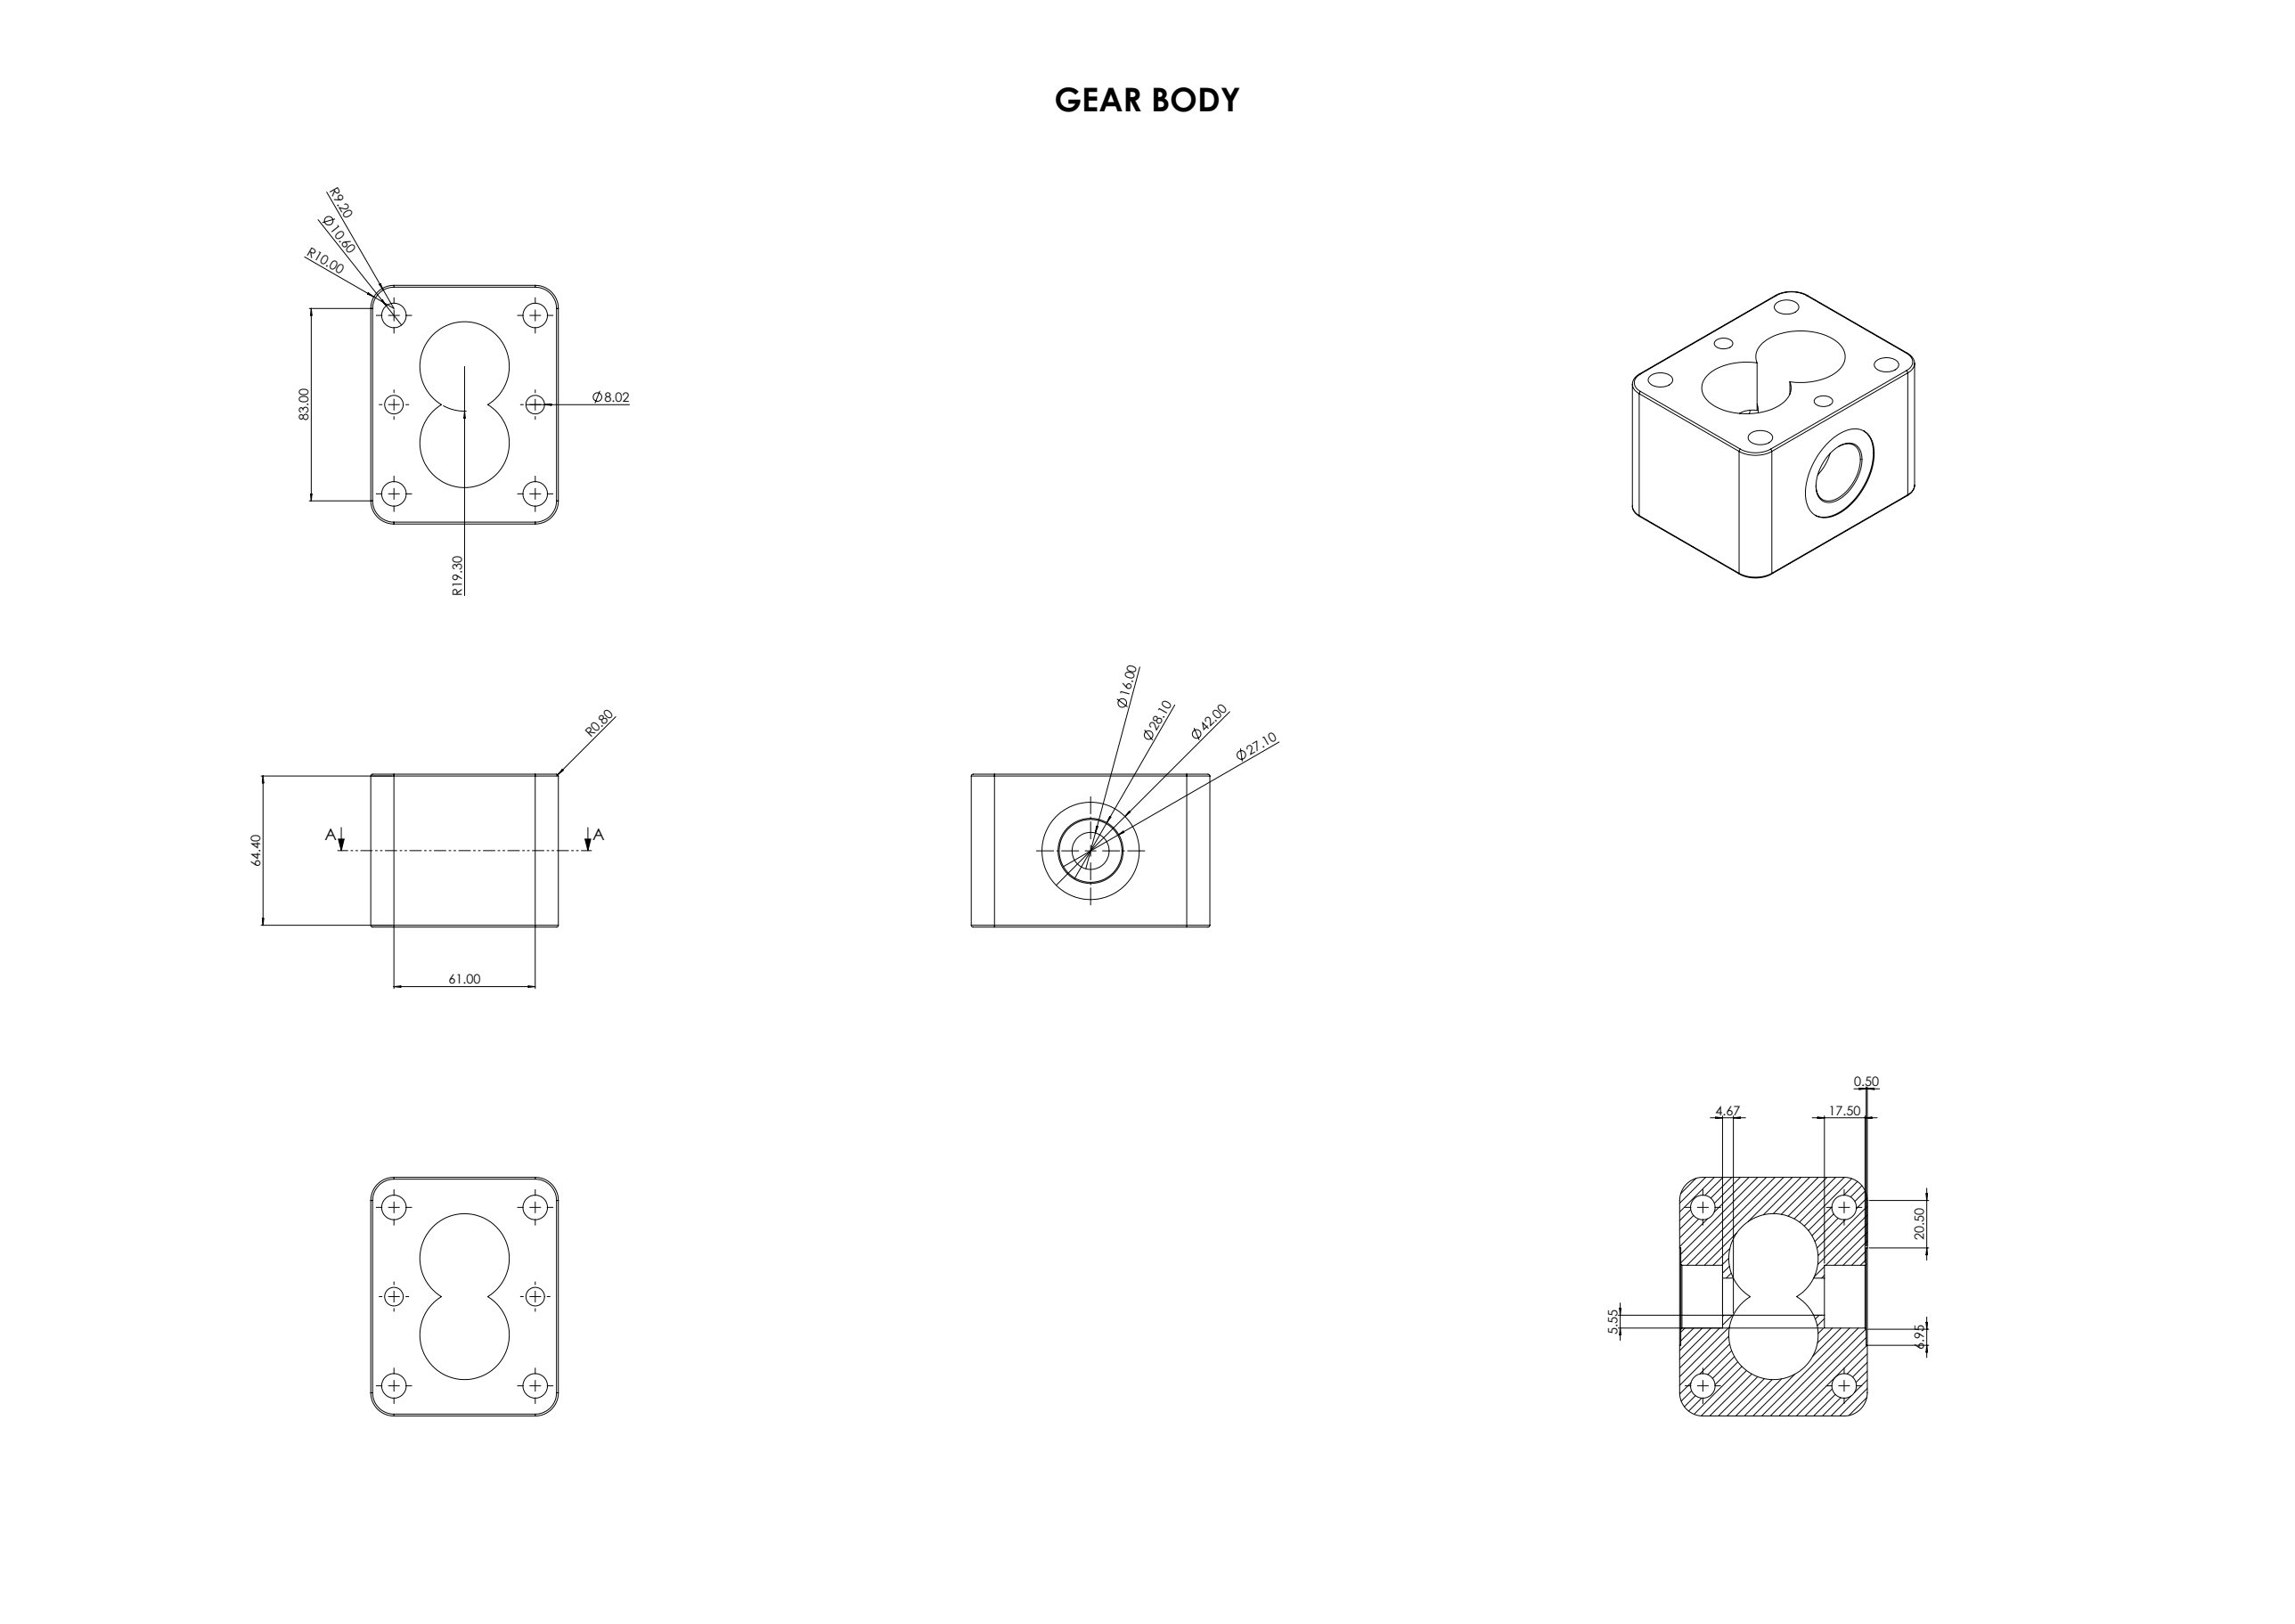
ISO-10303-21;
HEADER;
/* Generated by software containing ST-Developer
 * from STEP Tools, Inc. (www.steptools.com) 
 */

FILE_DESCRIPTION(
/* description */ (''),
/* implementation_level */ '2;1');

FILE_NAME(
/* name */ '02_Gear_Body.step',
/* time_stamp */ '2026-10-26T06:59:52-07:00',
/* author */ (''),
/* organization */ (''),
/* preprocessor_version */ 'ST-DEVELOPER v20.2',
/* originating_system */ 'Autodesk Translation Framework v15.15.0.0',
/* authorisation */ '');

FILE_SCHEMA (('AUTOMOTIVE_DESIGN { 1 0 10303 214 3 1 1 }'));
ENDSEC;

DATA;
#10=MECHANICAL_DESIGN_GEOMETRIC_PRESENTATION_REPRESENTATION('',(#165),#46395);
#137=SHAPE_REPRESENTATION_RELATIONSHIP('SRR','None',#46457,#151);
#151=ADVANCED_BREP_SHAPE_REPRESENTATION('',(#179),#46382);
#165=STYLED_ITEM('',(#46575),#179);
#179=MANIFOLD_SOLID_BREP('Body1',#24938);
#225=TOROIDAL_SURFACE('',#25463,9.19999999999999,0.8);
#226=TOROIDAL_SURFACE('',#25469,9.19999999999999,0.8);
#227=TOROIDAL_SURFACE('',#25475,9.2,0.8);
#228=TOROIDAL_SURFACE('',#25481,9.19999999999999,0.8);
#229=TOROIDAL_SURFACE('',#25503,9.19999999999999,0.8);
#230=TOROIDAL_SURFACE('',#25509,9.2,0.8);
#231=TOROIDAL_SURFACE('',#25515,9.19999999999999,0.8);
#232=TOROIDAL_SURFACE('',#25520,9.19999999999999,0.8);
#291=B_SPLINE_CURVE_WITH_KNOTS('',3,(#35527,#35528,#35529,#35530,#35531,
#35532,#35533,#35534,#35535,#35536,#35537,#35538,#35539,#35540),
 .UNSPECIFIED.,.F.,.F.,(4,2,2,2,2,2,4),(1.13912969187458,1.42739793020419,
1.87192783187775,2.07475703542203,2.27758623896631,2.45971948034335,2.64185272172039),
 .UNSPECIFIED.);
#292=B_SPLINE_CURVE_WITH_KNOTS('',3,(#35542,#35543,#35544,#35545,#35546,
#35547,#35548,#35549,#35550,#35551,#35552,#35553,#35554,#35555,#35556,#35557,
#35558,#35559,#35560,#35561,#35562,#35563,#35564,#35565,#35566,#35567),
 .UNSPECIFIED.,.F.,.F.,(4,2,2,2,2,2,2,2,2,2,2,2,4),(1.13912969187458,1.42739793020419,
1.87192783187775,2.07475703542203,2.27758623896631,2.45971948034335,2.64185272172039,
2.82398596309744,3.00611920447448,3.20894840801876,3.41177761156304,3.8563075132366,
4.14457575156621),.UNSPECIFIED.);
#293=B_SPLINE_CURVE_WITH_KNOTS('',3,(#35568,#35569,#35570,#35571,#35572,
#35573,#35574,#35575,#35576,#35577,#35578,#35579,#35580,#35581),
 .UNSPECIFIED.,.F.,.F.,(4,2,2,2,2,2,4),(2.64185272172039,2.82398596309744,
3.00611920447448,3.20894840801876,3.41177761156304,3.8563075132366,4.14457575156621),
 .UNSPECIFIED.);
#294=B_SPLINE_CURVE_WITH_KNOTS('',3,(#35587,#35588,#35589,#35590,#35591,
#35592,#35593,#35594,#35595,#35596,#35597,#35598,#35599,#35600),
 .UNSPECIFIED.,.F.,.F.,(4,2,2,2,2,2,4),(1.13912969187458,1.42739793020419,
1.87192783187775,2.07475703542203,2.27758623896631,2.45971948034335,2.64185272172039),
 .UNSPECIFIED.);
#295=B_SPLINE_CURVE_WITH_KNOTS('',3,(#35602,#35603,#35604,#35605,#35606,
#35607,#35608,#35609,#35610,#35611,#35612,#35613,#35614,#35615),
 .UNSPECIFIED.,.F.,.F.,(4,2,2,2,2,2,4),(2.64185272172039,2.82398596309744,
3.00611920447448,3.20894840801876,3.41177761156304,3.8563075132366,4.14457575156621),
 .UNSPECIFIED.);
#296=B_SPLINE_CURVE_WITH_KNOTS('',3,(#35627,#35628,#35629,#35630,#35631,
#35632,#35633,#35634,#35635,#35636,#35637,#35638,#35639,#35640,#35641,#35642,
#35643,#35644,#35645,#35646,#35647,#35648,#35649,#35650,#35651,#35652),
 .UNSPECIFIED.,.F.,.F.,(4,2,2,2,2,2,2,2,2,2,2,2,4),(1.13912969187458,1.42739793020419,
1.87192783187775,2.07475703542203,2.27758623896631,2.45971948034335,2.64185272172039,
2.82398596309744,3.00611920447448,3.20894840801876,3.41177761156304,3.8563075132366,
4.14457575156621),.UNSPECIFIED.);
#466=CYLINDRICAL_SURFACE('',#25449,13.55);
#467=CYLINDRICAL_SURFACE('',#25456,13.55);
#468=CYLINDRICAL_SURFACE('',#25460,0.8);
#469=CYLINDRICAL_SURFACE('',#25467,0.8);
#470=CYLINDRICAL_SURFACE('',#25473,0.8);
#471=CYLINDRICAL_SURFACE('',#25479,0.8);
#472=CYLINDRICAL_SURFACE('',#25484,9.99999999999999);
#473=CYLINDRICAL_SURFACE('',#25487,9.99999999999999);
#474=CYLINDRICAL_SURFACE('',#25500,0.8);
#475=CYLINDRICAL_SURFACE('',#25507,0.8);
#476=CYLINDRICAL_SURFACE('',#25513,0.8);
#477=CYLINDRICAL_SURFACE('',#25518,0.8);
#478=CYLINDRICAL_SURFACE('',#25522,10.);
#479=CYLINDRICAL_SURFACE('',#25524,9.99999999999999);
#480=CYLINDRICAL_SURFACE('',#25534,4.01);
#481=CYLINDRICAL_SURFACE('',#25537,4.01);
#482=CYLINDRICAL_SURFACE('',#25540,4.01);
#483=CYLINDRICAL_SURFACE('',#25543,4.01);
#484=CYLINDRICAL_SURFACE('',#25546,5.3);
#485=CYLINDRICAL_SURFACE('',#25547,5.3);
#486=CYLINDRICAL_SURFACE('',#25548,5.3);
#487=CYLINDRICAL_SURFACE('',#25549,5.3);
#488=CYLINDRICAL_SURFACE('',#25550,8.);
#489=CYLINDRICAL_SURFACE('',#25552,19.3);
#490=CYLINDRICAL_SURFACE('',#25554,21.);
#491=CYLINDRICAL_SURFACE('',#25556,8.);
#492=CYLINDRICAL_SURFACE('',#25558,19.3);
#493=CYLINDRICAL_SURFACE('',#25560,21.);
#611=FACE_BOUND('',#3282,.T.);
#612=FACE_BOUND('',#3286,.T.);
#613=FACE_BOUND('',#3299,.T.);
#614=FACE_BOUND('',#3301,.T.);
#615=FACE_BOUND('',#3302,.T.);
#616=FACE_BOUND('',#3303,.T.);
#617=FACE_BOUND('',#3304,.T.);
#618=FACE_BOUND('',#3305,.T.);
#619=FACE_BOUND('',#3306,.T.);
#620=FACE_BOUND('',#3307,.T.);
#621=FACE_BOUND('',#3320,.T.);
#622=FACE_BOUND('',#3321,.T.);
#623=FACE_BOUND('',#3322,.T.);
#624=FACE_BOUND('',#3323,.T.);
#625=FACE_BOUND('',#3324,.T.);
#626=FACE_BOUND('',#3325,.T.);
#627=FACE_BOUND('',#3326,.T.);
#628=FACE_BOUND('',#3342,.T.);
#629=FACE_BOUND('',#3347,.T.);
#630=FACE_BOUND('',#3350,.T.);
#764=PLANE('',#25451);
#765=PLANE('',#25458);
#766=PLANE('',#25486);
#767=PLANE('',#25489);
#768=PLANE('',#25491);
#769=PLANE('',#25523);
#770=PLANE('',#25525);
#771=PLANE('',#25536);
#772=PLANE('',#25539);
#773=PLANE('',#25542);
#774=PLANE('',#25545);
#775=PLANE('',#25553);
#776=PLANE('',#25559);
#777=PLANE('',#25561);
#1923=FACE_OUTER_BOUND('',#3279,.T.);
#1924=FACE_OUTER_BOUND('',#3280,.T.);
#1925=FACE_OUTER_BOUND('',#3281,.T.);
#1926=FACE_OUTER_BOUND('',#3283,.T.);
#1927=FACE_OUTER_BOUND('',#3284,.T.);
#1928=FACE_OUTER_BOUND('',#3285,.T.);
#1929=FACE_OUTER_BOUND('',#3287,.T.);
#1930=FACE_OUTER_BOUND('',#3288,.T.);
#1931=FACE_OUTER_BOUND('',#3289,.T.);
#1932=FACE_OUTER_BOUND('',#3290,.T.);
#1933=FACE_OUTER_BOUND('',#3291,.T.);
#1934=FACE_OUTER_BOUND('',#3292,.T.);
#1935=FACE_OUTER_BOUND('',#3293,.T.);
#1936=FACE_OUTER_BOUND('',#3294,.T.);
#1937=FACE_OUTER_BOUND('',#3295,.T.);
#1938=FACE_OUTER_BOUND('',#3296,.T.);
#1939=FACE_OUTER_BOUND('',#3297,.T.);
#1940=FACE_OUTER_BOUND('',#3298,.T.);
#1941=FACE_OUTER_BOUND('',#3300,.T.);
#1942=FACE_OUTER_BOUND('',#3308,.T.);
#1943=FACE_OUTER_BOUND('',#3309,.T.);
#1944=FACE_OUTER_BOUND('',#3310,.T.);
#1945=FACE_OUTER_BOUND('',#3311,.T.);
#1946=FACE_OUTER_BOUND('',#3312,.T.);
#1947=FACE_OUTER_BOUND('',#3313,.T.);
#1948=FACE_OUTER_BOUND('',#3314,.T.);
#1949=FACE_OUTER_BOUND('',#3315,.T.);
#1950=FACE_OUTER_BOUND('',#3316,.T.);
#1951=FACE_OUTER_BOUND('',#3317,.T.);
#1952=FACE_OUTER_BOUND('',#3318,.T.);
#1953=FACE_OUTER_BOUND('',#3319,.T.);
#1954=FACE_OUTER_BOUND('',#3327,.T.);
#1955=FACE_OUTER_BOUND('',#3328,.T.);
#1956=FACE_OUTER_BOUND('',#3329,.T.);
#1957=FACE_OUTER_BOUND('',#3330,.T.);
#1958=FACE_OUTER_BOUND('',#3331,.T.);
#1959=FACE_OUTER_BOUND('',#3332,.T.);
#1960=FACE_OUTER_BOUND('',#3333,.T.);
#1961=FACE_OUTER_BOUND('',#3334,.T.);
#1962=FACE_OUTER_BOUND('',#3335,.T.);
#1963=FACE_OUTER_BOUND('',#3336,.T.);
#1964=FACE_OUTER_BOUND('',#3337,.T.);
#1965=FACE_OUTER_BOUND('',#3338,.T.);
#1966=FACE_OUTER_BOUND('',#3339,.T.);
#1967=FACE_OUTER_BOUND('',#3340,.T.);
#1968=FACE_OUTER_BOUND('',#3341,.T.);
#1969=FACE_OUTER_BOUND('',#3343,.T.);
#1970=FACE_OUTER_BOUND('',#3344,.T.);
#1971=FACE_OUTER_BOUND('',#3345,.T.);
#1972=FACE_OUTER_BOUND('',#3346,.T.);
#1973=FACE_OUTER_BOUND('',#3348,.T.);
#1974=FACE_OUTER_BOUND('',#3349,.T.);
#3279=EDGE_LOOP('',(#17354,#17355,#17356,#17357));
#3280=EDGE_LOOP('',(#17358,#17359,#17360,#17361));
#3281=EDGE_LOOP('',(#17362));
#3282=EDGE_LOOP('',(#17363));
#3283=EDGE_LOOP('',(#17364,#17365,#17366,#17367));
#3284=EDGE_LOOP('',(#17368,#17369,#17370,#17371));
#3285=EDGE_LOOP('',(#17372));
#3286=EDGE_LOOP('',(#17373));
#3287=EDGE_LOOP('',(#17374,#17375,#17376,#17377));
#3288=EDGE_LOOP('',(#17378,#17379,#17380,#17381));
#3289=EDGE_LOOP('',(#17382,#17383,#17384,#17385));
#3290=EDGE_LOOP('',(#17386,#17387,#17388,#17389));
#3291=EDGE_LOOP('',(#17390,#17391,#17392,#17393));
#3292=EDGE_LOOP('',(#17394,#17395,#17396,#17397));
#3293=EDGE_LOOP('',(#17398,#17399,#17400,#17401));
#3294=EDGE_LOOP('',(#17402,#17403,#17404,#17405));
#3295=EDGE_LOOP('',(#17406,#17407,#17408,#17409));
#3296=EDGE_LOOP('',(#17410,#17411,#17412,#17413));
#3297=EDGE_LOOP('',(#17414,#17415,#17416,#17417));
#3298=EDGE_LOOP('',(#17418,#17419,#17420,#17421));
#3299=EDGE_LOOP('',(#17422));
#3300=EDGE_LOOP('',(#17423,#17424,#17425,#17426,#17427,#17428,#17429,#17430));
#3301=EDGE_LOOP('',(#17431));
#3302=EDGE_LOOP('',(#17432));
#3303=EDGE_LOOP('',(#17433,#17434));
#3304=EDGE_LOOP('',(#17435));
#3305=EDGE_LOOP('',(#17436));
#3306=EDGE_LOOP('',(#17437));
#3307=EDGE_LOOP('',(#17438));
#3308=EDGE_LOOP('',(#17439,#17440,#17441,#17442));
#3309=EDGE_LOOP('',(#17443,#17444,#17445,#17446));
#3310=EDGE_LOOP('',(#17447,#17448,#17449,#17450));
#3311=EDGE_LOOP('',(#17451,#17452,#17453,#17454));
#3312=EDGE_LOOP('',(#17455,#17456,#17457,#17458));
#3313=EDGE_LOOP('',(#17459,#17460,#17461,#17462));
#3314=EDGE_LOOP('',(#17463,#17464,#17465,#17466));
#3315=EDGE_LOOP('',(#17467,#17468,#17469,#17470));
#3316=EDGE_LOOP('',(#17471,#17472,#17473,#17474));
#3317=EDGE_LOOP('',(#17475,#17476,#17477,#17478));
#3318=EDGE_LOOP('',(#17479,#17480,#17481,#17482));
#3319=EDGE_LOOP('',(#17483,#17484,#17485,#17486,#17487,#17488,#17489,#17490));
#3320=EDGE_LOOP('',(#17491));
#3321=EDGE_LOOP('',(#17492));
#3322=EDGE_LOOP('',(#17493,#17494));
#3323=EDGE_LOOP('',(#17495));
#3324=EDGE_LOOP('',(#17496));
#3325=EDGE_LOOP('',(#17497));
#3326=EDGE_LOOP('',(#17498));
#3327=EDGE_LOOP('',(#17499,#17500,#17501,#17502));
#3328=EDGE_LOOP('',(#17503));
#3329=EDGE_LOOP('',(#17504,#17505,#17506,#17507));
#3330=EDGE_LOOP('',(#17508));
#3331=EDGE_LOOP('',(#17509,#17510,#17511,#17512));
#3332=EDGE_LOOP('',(#17513));
#3333=EDGE_LOOP('',(#17514,#17515,#17516,#17517));
#3334=EDGE_LOOP('',(#17518));
#3335=EDGE_LOOP('',(#17519,#17520,#17521,#17522));
#3336=EDGE_LOOP('',(#17523,#17524,#17525,#17526));
#3337=EDGE_LOOP('',(#17527,#17528,#17529,#17530));
#3338=EDGE_LOOP('',(#17531,#17532,#17533,#17534));
#3339=EDGE_LOOP('',(#17535,#17536,#17537,#17538,#17539,#17540));
#3340=EDGE_LOOP('',(#17541,#17542,#17543,#17544,#17545,#17546,#17547,#17548,
#17549,#17550));
#3341=EDGE_LOOP('',(#17551));
#3342=EDGE_LOOP('',(#17552));
#3343=EDGE_LOOP('',(#17553,#17554,#17555,#17556));
#3344=EDGE_LOOP('',(#17557,#17558,#17559,#17560,#17561,#17562));
#3345=EDGE_LOOP('',(#17563,#17564,#17565,#17566,#17567,#17568,#17569,#17570));
#3346=EDGE_LOOP('',(#17571));
#3347=EDGE_LOOP('',(#17572));
#3348=EDGE_LOOP('',(#17573,#17574,#17575,#17576));
#3349=EDGE_LOOP('',(#17577,#17578,#17579,#17580));
#3350=EDGE_LOOP('',(#17581));
#4722=LINE('',#35324,#7591);
#4723=LINE('',#35328,#7592);
#4724=LINE('',#35337,#7593);
#4725=LINE('',#35341,#7594);
#4726=LINE('',#35351,#7595);
#4727=LINE('',#35354,#7596);
#4728=LINE('',#35365,#7597);
#4729=LINE('',#35366,#7598);
#4730=LINE('',#35377,#7599);
#4731=LINE('',#35378,#7600);
#4732=LINE('',#35389,#7601);
#4733=LINE('',#35390,#7602);
#4734=LINE('',#35396,#7603);
#4735=LINE('',#35399,#7604);
#4736=LINE('',#35402,#7605);
#4737=LINE('',#35403,#7606);
#4738=LINE('',#35406,#7607);
#4739=LINE('',#35410,#7608);
#4740=LINE('',#35411,#7609);
#4741=LINE('',#35436,#7610);
#4742=LINE('',#35447,#7611);
#4743=LINE('',#35448,#7612);
#4744=LINE('',#35458,#7613);
#4745=LINE('',#35459,#7614);
#4746=LINE('',#35467,#7615);
#4747=LINE('',#35471,#7616);
#4748=LINE('',#35472,#7617);
#4749=LINE('',#35474,#7618);
#4750=LINE('',#35495,#7619);
#4751=LINE('',#35500,#7620);
#4752=LINE('',#35505,#7621);
#4753=LINE('',#35510,#7622);
#4754=LINE('',#35514,#7623);
#4755=LINE('',#35516,#7624);
#4756=LINE('',#35518,#7625);
#4757=LINE('',#35520,#7626);
#4758=LINE('',#35525,#7627);
#4759=LINE('',#35583,#7628);
#4760=LINE('',#35585,#7629);
#4761=LINE('',#35616,#7630);
#4762=LINE('',#35617,#7631);
#4763=LINE('',#35622,#7632);
#4764=LINE('',#35626,#7633);
#4765=LINE('',#35656,#7634);
#7591=VECTOR('',#27805,13.8);
#7592=VECTOR('',#27810,13.55);
#7593=VECTOR('',#27821,13.8);
#7594=VECTOR('',#27826,13.55);
#7595=VECTOR('',#27837,10.);
#7596=VECTOR('',#27840,10.);
#7597=VECTOR('',#27853,10.);
#7598=VECTOR('',#27854,10.);
#7599=VECTOR('',#27867,10.);
#7600=VECTOR('',#27868,10.);
#7601=VECTOR('',#27881,10.);
#7602=VECTOR('',#27882,10.);
#7603=VECTOR('',#27891,10.);
#7604=VECTOR('',#27894,10.);
#7605=VECTOR('',#27897,10.);
#7606=VECTOR('',#27898,10.);
#7607=VECTOR('',#27901,10.);
#7608=VECTOR('',#27906,10.);
#7609=VECTOR('',#27907,10.);
#7610=VECTOR('',#27934,10.);
#7611=VECTOR('',#27947,10.);
#7612=VECTOR('',#27948,10.);
#7613=VECTOR('',#27961,10.);
#7614=VECTOR('',#27962,10.);
#7615=VECTOR('',#27973,10.);
#7616=VECTOR('',#27980,10.);
#7617=VECTOR('',#27981,10.);
#7618=VECTOR('',#27984,10.);
#7619=VECTOR('',#28007,4.01);
#7620=VECTOR('',#28014,4.01);
#7621=VECTOR('',#28021,4.01);
#7622=VECTOR('',#28028,4.01);
#7623=VECTOR('',#28035,5.3);
#7624=VECTOR('',#28038,5.3);
#7625=VECTOR('',#28041,5.3);
#7626=VECTOR('',#28044,5.3);
#7627=VECTOR('',#28049,8.);
#7628=VECTOR('',#28052,10.);
#7629=VECTOR('',#28053,10.);
#7630=VECTOR('',#28054,10.);
#7631=VECTOR('',#28055,10.);
#7632=VECTOR('',#28062,21.);
#7633=VECTOR('',#28067,8.);
#7634=VECTOR('',#28074,21.);
#10441=CIRCLE('',#25447,14.05);
#10442=CIRCLE('',#25448,13.55);
#10443=CIRCLE('',#25450,13.55);
#10444=CIRCLE('',#25452,21.);
#10445=CIRCLE('',#25454,14.05);
#10446=CIRCLE('',#25455,13.55);
#10447=CIRCLE('',#25457,13.55);
#10448=CIRCLE('',#25459,21.);
#10449=CIRCLE('',#25461,0.800000000000001);
#10450=CIRCLE('',#25462,0.800000000000001);
#10451=CIRCLE('',#25464,0.799999999999992);
#10452=CIRCLE('',#25465,9.19999999999999);
#10453=CIRCLE('',#25466,9.99999999999999);
#10454=CIRCLE('',#25468,0.800000000000001);
#10455=CIRCLE('',#25470,0.800000000000005);
#10456=CIRCLE('',#25471,9.19999999999999);
#10457=CIRCLE('',#25472,9.99999999999999);
#10458=CIRCLE('',#25474,0.800000000000001);
#10459=CIRCLE('',#25476,0.800000000000001);
#10460=CIRCLE('',#25477,9.2);
#10461=CIRCLE('',#25478,9.99999999999999);
#10462=CIRCLE('',#25480,0.800000000000001);
#10463=CIRCLE('',#25482,9.19999999999999);
#10464=CIRCLE('',#25483,9.99999999999999);
#10465=CIRCLE('',#25485,9.99999999999999);
#10466=CIRCLE('',#25488,9.99999999999999);
#10467=CIRCLE('',#25490,21.);
#10468=CIRCLE('',#25492,4.01);
#10469=CIRCLE('',#25493,4.01);
#10470=CIRCLE('',#25494,19.3);
#10471=CIRCLE('',#25495,19.3);
#10472=CIRCLE('',#25496,5.3);
#10473=CIRCLE('',#25497,5.3);
#10474=CIRCLE('',#25498,5.3);
#10475=CIRCLE('',#25499,5.3);
#10476=CIRCLE('',#25501,0.800000000000001);
#10477=CIRCLE('',#25502,0.799999999999992);
#10478=CIRCLE('',#25504,0.800000000000001);
#10479=CIRCLE('',#25505,9.19999999999999);
#10480=CIRCLE('',#25506,9.99999999999999);
#10481=CIRCLE('',#25508,0.800000000000005);
#10482=CIRCLE('',#25510,0.799999999999996);
#10483=CIRCLE('',#25511,9.2);
#10484=CIRCLE('',#25512,9.99999999999999);
#10485=CIRCLE('',#25514,0.80000000000001);
#10486=CIRCLE('',#25516,0.800000000000001);
#10487=CIRCLE('',#25517,9.19999999999999);
#10488=CIRCLE('',#25519,0.799999999999992);
#10489=CIRCLE('',#25521,9.19999999999999);
#10490=CIRCLE('',#25526,4.01);
#10491=CIRCLE('',#25527,4.01);
#10492=CIRCLE('',#25528,19.3);
#10493=CIRCLE('',#25529,19.3);
#10494=CIRCLE('',#25530,5.3);
#10495=CIRCLE('',#25531,5.3);
#10496=CIRCLE('',#25532,5.3);
#10497=CIRCLE('',#25533,5.3);
#10498=CIRCLE('',#25535,4.01);
#10499=CIRCLE('',#25538,4.01);
#10500=CIRCLE('',#25541,4.01);
#10501=CIRCLE('',#25544,4.01);
#10502=CIRCLE('',#25551,8.);
#10503=CIRCLE('',#25555,21.);
#10504=CIRCLE('',#25557,8.);
#10984=VERTEX_POINT('',#35321);
#10985=VERTEX_POINT('',#35323);
#10986=VERTEX_POINT('',#35327);
#10987=VERTEX_POINT('',#35331);
#10988=VERTEX_POINT('',#35334);
#10989=VERTEX_POINT('',#35336);
#10990=VERTEX_POINT('',#35340);
#10991=VERTEX_POINT('',#35344);
#10992=VERTEX_POINT('',#35347);
#10993=VERTEX_POINT('',#35348);
#10994=VERTEX_POINT('',#35350);
#10995=VERTEX_POINT('',#35352);
#10996=VERTEX_POINT('',#35356);
#10997=VERTEX_POINT('',#35357);
#10998=VERTEX_POINT('',#35362);
#10999=VERTEX_POINT('',#35363);
#11000=VERTEX_POINT('',#35368);
#11001=VERTEX_POINT('',#35369);
#11002=VERTEX_POINT('',#35374);
#11003=VERTEX_POINT('',#35375);
#11004=VERTEX_POINT('',#35380);
#11005=VERTEX_POINT('',#35381);
#11006=VERTEX_POINT('',#35386);
#11007=VERTEX_POINT('',#35387);
#11008=VERTEX_POINT('',#35395);
#11009=VERTEX_POINT('',#35397);
#11010=VERTEX_POINT('',#35401);
#11011=VERTEX_POINT('',#35405);
#11012=VERTEX_POINT('',#35409);
#11013=VERTEX_POINT('',#35412);
#11014=VERTEX_POINT('',#35415);
#11015=VERTEX_POINT('',#35417);
#11016=VERTEX_POINT('',#35419);
#11017=VERTEX_POINT('',#35420);
#11018=VERTEX_POINT('',#35423);
#11019=VERTEX_POINT('',#35425);
#11020=VERTEX_POINT('',#35427);
#11021=VERTEX_POINT('',#35429);
#11022=VERTEX_POINT('',#35432);
#11023=VERTEX_POINT('',#35434);
#11024=VERTEX_POINT('',#35438);
#11025=VERTEX_POINT('',#35439);
#11026=VERTEX_POINT('',#35444);
#11027=VERTEX_POINT('',#35445);
#11028=VERTEX_POINT('',#35450);
#11029=VERTEX_POINT('',#35451);
#11030=VERTEX_POINT('',#35456);
#11031=VERTEX_POINT('',#35461);
#11032=VERTEX_POINT('',#35465);
#11033=VERTEX_POINT('',#35477);
#11034=VERTEX_POINT('',#35479);
#11035=VERTEX_POINT('',#35481);
#11036=VERTEX_POINT('',#35482);
#11037=VERTEX_POINT('',#35485);
#11038=VERTEX_POINT('',#35487);
#11039=VERTEX_POINT('',#35489);
#11040=VERTEX_POINT('',#35491);
#11041=VERTEX_POINT('',#35494);
#11042=VERTEX_POINT('',#35499);
#11043=VERTEX_POINT('',#35504);
#11044=VERTEX_POINT('',#35509);
#11045=VERTEX_POINT('',#35522);
#11046=VERTEX_POINT('',#35524);
#11047=VERTEX_POINT('',#35526);
#11048=VERTEX_POINT('',#35541);
#11049=VERTEX_POINT('',#35584);
#11050=VERTEX_POINT('',#35586);
#11051=VERTEX_POINT('',#35601);
#11052=VERTEX_POINT('',#35620);
#11053=VERTEX_POINT('',#35624);
#13430=EDGE_CURVE('',#10984,#10984,#10441,.T.);
#13431=EDGE_CURVE('',#10984,#10985,#4722,.T.);
#13432=EDGE_CURVE('',#10985,#10985,#10442,.T.);
#13433=EDGE_CURVE('',#10985,#10986,#4723,.T.);
#13434=EDGE_CURVE('',#10986,#10986,#10443,.T.);
#13435=EDGE_CURVE('',#10987,#10987,#10444,.T.);
#13436=EDGE_CURVE('',#10988,#10988,#10445,.T.);
#13437=EDGE_CURVE('',#10988,#10989,#4724,.T.);
#13438=EDGE_CURVE('',#10989,#10989,#10446,.T.);
#13439=EDGE_CURVE('',#10989,#10990,#4725,.T.);
#13440=EDGE_CURVE('',#10990,#10990,#10447,.T.);
#13441=EDGE_CURVE('',#10991,#10991,#10448,.T.);
#13442=EDGE_CURVE('',#10992,#10993,#10449,.T.);
#13443=EDGE_CURVE('',#10993,#10994,#4726,.T.);
#13444=EDGE_CURVE('',#10994,#10995,#10450,.T.);
#13445=EDGE_CURVE('',#10995,#10992,#4727,.T.);
#13446=EDGE_CURVE('',#10996,#10997,#10451,.T.);
#13447=EDGE_CURVE('',#10997,#10995,#10452,.T.);
#13448=EDGE_CURVE('',#10994,#10996,#10453,.T.);
#13449=EDGE_CURVE('',#10998,#10999,#10454,.T.);
#13450=EDGE_CURVE('',#10999,#10997,#4728,.T.);
#13451=EDGE_CURVE('',#10996,#10998,#4729,.T.);
#13452=EDGE_CURVE('',#11000,#11001,#10455,.T.);
#13453=EDGE_CURVE('',#11001,#10999,#10456,.T.);
#13454=EDGE_CURVE('',#10998,#11000,#10457,.T.);
#13455=EDGE_CURVE('',#11002,#11003,#10458,.T.);
#13456=EDGE_CURVE('',#11003,#11001,#4730,.T.);
#13457=EDGE_CURVE('',#11000,#11002,#4731,.T.);
#13458=EDGE_CURVE('',#11004,#11005,#10459,.T.);
#13459=EDGE_CURVE('',#11005,#11003,#10460,.T.);
#13460=EDGE_CURVE('',#11002,#11004,#10461,.T.);
#13461=EDGE_CURVE('',#11006,#11007,#10462,.T.);
#13462=EDGE_CURVE('',#11007,#11005,#4732,.T.);
#13463=EDGE_CURVE('',#11004,#11006,#4733,.T.);
#13464=EDGE_CURVE('',#10992,#11007,#10463,.T.);
#13465=EDGE_CURVE('',#11006,#10993,#10464,.T.);
#13466=EDGE_CURVE('',#11008,#10998,#4734,.T.);
#13467=EDGE_CURVE('',#11009,#11008,#10465,.T.);
#13468=EDGE_CURVE('',#11009,#11000,#4735,.T.);
#13469=EDGE_CURVE('',#11010,#10996,#4736,.T.);
#13470=EDGE_CURVE('',#11008,#11010,#4737,.T.);
#13471=EDGE_CURVE('',#11011,#10994,#4738,.T.);
#13472=EDGE_CURVE('',#11010,#11011,#10466,.T.);
#13473=EDGE_CURVE('',#11012,#10993,#4739,.T.);
#13474=EDGE_CURVE('',#11011,#11012,#4740,.T.);
#13475=EDGE_CURVE('',#11013,#11013,#10467,.T.);
#13476=EDGE_CURVE('',#11014,#11014,#10468,.T.);
#13477=EDGE_CURVE('',#11015,#11015,#10469,.T.);
#13478=EDGE_CURVE('',#11016,#11017,#10470,.T.);
#13479=EDGE_CURVE('',#11017,#11016,#10471,.T.);
#13480=EDGE_CURVE('',#11018,#11018,#10472,.T.);
#13481=EDGE_CURVE('',#11019,#11019,#10473,.T.);
#13482=EDGE_CURVE('',#11020,#11020,#10474,.T.);
#13483=EDGE_CURVE('',#11021,#11021,#10475,.T.);
#13484=EDGE_CURVE('',#11022,#11011,#10476,.T.);
#13485=EDGE_CURVE('',#11012,#11023,#10477,.T.);
#13486=EDGE_CURVE('',#11023,#11022,#4741,.T.);
#13487=EDGE_CURVE('',#11024,#11025,#10478,.T.);
#13488=EDGE_CURVE('',#11025,#11023,#10479,.T.);
#13489=EDGE_CURVE('',#11012,#11024,#10480,.T.);
#13490=EDGE_CURVE('',#11026,#11027,#10481,.T.);
#13491=EDGE_CURVE('',#11027,#11025,#4742,.T.);
#13492=EDGE_CURVE('',#11024,#11026,#4743,.T.);
#13493=EDGE_CURVE('',#11028,#11029,#10482,.T.);
#13494=EDGE_CURVE('',#11029,#11027,#10483,.T.);
#13495=EDGE_CURVE('',#11026,#11028,#10484,.T.);
#13496=EDGE_CURVE('',#11009,#11030,#10485,.T.);
#13497=EDGE_CURVE('',#11030,#11029,#4744,.T.);
#13498=EDGE_CURVE('',#11028,#11009,#4745,.T.);
#13499=EDGE_CURVE('',#11008,#11031,#10486,.T.);
#13500=EDGE_CURVE('',#11031,#11030,#10487,.T.);
#13501=EDGE_CURVE('',#11010,#11032,#10488,.T.);
#13502=EDGE_CURVE('',#11032,#11031,#4746,.T.);
#13503=EDGE_CURVE('',#11022,#11032,#10489,.T.);
#13504=EDGE_CURVE('',#11028,#11002,#4747,.T.);
#13505=EDGE_CURVE('',#11026,#11004,#4748,.T.);
#13506=EDGE_CURVE('',#11024,#11006,#4749,.T.);
#13507=EDGE_CURVE('',#11033,#11033,#10490,.T.);
#13508=EDGE_CURVE('',#11034,#11034,#10491,.T.);
#13509=EDGE_CURVE('',#11035,#11036,#10492,.T.);
#13510=EDGE_CURVE('',#11036,#11035,#10493,.T.);
#13511=EDGE_CURVE('',#11037,#11037,#10494,.T.);
#13512=EDGE_CURVE('',#11038,#11038,#10495,.T.);
#13513=EDGE_CURVE('',#11039,#11039,#10496,.T.);
#13514=EDGE_CURVE('',#11040,#11040,#10497,.T.);
#13515=EDGE_CURVE('',#11014,#11041,#4750,.T.);
#13516=EDGE_CURVE('',#11041,#11041,#10498,.T.);
#13517=EDGE_CURVE('',#11015,#11042,#4751,.T.);
#13518=EDGE_CURVE('',#11042,#11042,#10499,.T.);
#13519=EDGE_CURVE('',#11033,#11043,#4752,.T.);
#13520=EDGE_CURVE('',#11043,#11043,#10500,.T.);
#13521=EDGE_CURVE('',#11034,#11044,#4753,.T.);
#13522=EDGE_CURVE('',#11044,#11044,#10501,.T.);
#13523=EDGE_CURVE('',#11040,#11021,#4754,.T.);
#13524=EDGE_CURVE('',#11039,#11020,#4755,.T.);
#13525=EDGE_CURVE('',#11038,#11019,#4756,.T.);
#13526=EDGE_CURVE('',#11037,#11018,#4757,.T.);
#13527=EDGE_CURVE('',#11045,#11045,#10502,.T.);
#13528=EDGE_CURVE('',#11045,#11046,#4758,.T.);
#13529=EDGE_CURVE('',#11047,#11046,#291,.T.);
#13530=EDGE_CURVE('',#11048,#11047,#292,.T.);
#13531=EDGE_CURVE('',#11046,#11048,#293,.T.);
#13532=EDGE_CURVE('',#11048,#11017,#4759,.T.);
#13533=EDGE_CURVE('',#11049,#11016,#4760,.T.);
#13534=EDGE_CURVE('',#11049,#11050,#294,.T.);
#13535=EDGE_CURVE('',#11050,#11051,#295,.T.);
#13536=EDGE_CURVE('',#11036,#11051,#4761,.T.);
#13537=EDGE_CURVE('',#11035,#11047,#4762,.T.);
#13538=EDGE_CURVE('',#11052,#11052,#10503,.T.);
#13539=EDGE_CURVE('',#11052,#10991,#4763,.T.);
#13540=EDGE_CURVE('',#11053,#11053,#10504,.T.);
#13541=EDGE_CURVE('',#11053,#11050,#4764,.T.);
#13542=EDGE_CURVE('',#11051,#11049,#296,.T.);
#13543=EDGE_CURVE('',#11013,#10987,#4765,.T.);
#17354=ORIENTED_EDGE('',*,*,#13430,.T.);
#17355=ORIENTED_EDGE('',*,*,#13431,.T.);
#17356=ORIENTED_EDGE('',*,*,#13432,.T.);
#17357=ORIENTED_EDGE('',*,*,#13431,.F.);
#17358=ORIENTED_EDGE('',*,*,#13432,.F.);
#17359=ORIENTED_EDGE('',*,*,#13433,.T.);
#17360=ORIENTED_EDGE('',*,*,#13434,.T.);
#17361=ORIENTED_EDGE('',*,*,#13433,.F.);
#17362=ORIENTED_EDGE('',*,*,#13435,.F.);
#17363=ORIENTED_EDGE('',*,*,#13430,.F.);
#17364=ORIENTED_EDGE('',*,*,#13436,.T.);
#17365=ORIENTED_EDGE('',*,*,#13437,.T.);
#17366=ORIENTED_EDGE('',*,*,#13438,.T.);
#17367=ORIENTED_EDGE('',*,*,#13437,.F.);
#17368=ORIENTED_EDGE('',*,*,#13438,.F.);
#17369=ORIENTED_EDGE('',*,*,#13439,.T.);
#17370=ORIENTED_EDGE('',*,*,#13440,.T.);
#17371=ORIENTED_EDGE('',*,*,#13439,.F.);
#17372=ORIENTED_EDGE('',*,*,#13441,.F.);
#17373=ORIENTED_EDGE('',*,*,#13436,.F.);
#17374=ORIENTED_EDGE('',*,*,#13442,.T.);
#17375=ORIENTED_EDGE('',*,*,#13443,.T.);
#17376=ORIENTED_EDGE('',*,*,#13444,.T.);
#17377=ORIENTED_EDGE('',*,*,#13445,.T.);
#17378=ORIENTED_EDGE('',*,*,#13446,.T.);
#17379=ORIENTED_EDGE('',*,*,#13447,.T.);
#17380=ORIENTED_EDGE('',*,*,#13444,.F.);
#17381=ORIENTED_EDGE('',*,*,#13448,.T.);
#17382=ORIENTED_EDGE('',*,*,#13449,.T.);
#17383=ORIENTED_EDGE('',*,*,#13450,.T.);
#17384=ORIENTED_EDGE('',*,*,#13446,.F.);
#17385=ORIENTED_EDGE('',*,*,#13451,.T.);
#17386=ORIENTED_EDGE('',*,*,#13452,.T.);
#17387=ORIENTED_EDGE('',*,*,#13453,.T.);
#17388=ORIENTED_EDGE('',*,*,#13449,.F.);
#17389=ORIENTED_EDGE('',*,*,#13454,.T.);
#17390=ORIENTED_EDGE('',*,*,#13455,.T.);
#17391=ORIENTED_EDGE('',*,*,#13456,.T.);
#17392=ORIENTED_EDGE('',*,*,#13452,.F.);
#17393=ORIENTED_EDGE('',*,*,#13457,.T.);
#17394=ORIENTED_EDGE('',*,*,#13458,.T.);
#17395=ORIENTED_EDGE('',*,*,#13459,.T.);
#17396=ORIENTED_EDGE('',*,*,#13455,.F.);
#17397=ORIENTED_EDGE('',*,*,#13460,.T.);
#17398=ORIENTED_EDGE('',*,*,#13461,.T.);
#17399=ORIENTED_EDGE('',*,*,#13462,.T.);
#17400=ORIENTED_EDGE('',*,*,#13458,.F.);
#17401=ORIENTED_EDGE('',*,*,#13463,.T.);
#17402=ORIENTED_EDGE('',*,*,#13442,.F.);
#17403=ORIENTED_EDGE('',*,*,#13464,.T.);
#17404=ORIENTED_EDGE('',*,*,#13461,.F.);
#17405=ORIENTED_EDGE('',*,*,#13465,.T.);
#17406=ORIENTED_EDGE('',*,*,#13454,.F.);
#17407=ORIENTED_EDGE('',*,*,#13466,.F.);
#17408=ORIENTED_EDGE('',*,*,#13467,.F.);
#17409=ORIENTED_EDGE('',*,*,#13468,.T.);
#17410=ORIENTED_EDGE('',*,*,#13451,.F.);
#17411=ORIENTED_EDGE('',*,*,#13469,.F.);
#17412=ORIENTED_EDGE('',*,*,#13470,.F.);
#17413=ORIENTED_EDGE('',*,*,#13466,.T.);
#17414=ORIENTED_EDGE('',*,*,#13448,.F.);
#17415=ORIENTED_EDGE('',*,*,#13471,.F.);
#17416=ORIENTED_EDGE('',*,*,#13472,.F.);
#17417=ORIENTED_EDGE('',*,*,#13469,.T.);
#17418=ORIENTED_EDGE('',*,*,#13443,.F.);
#17419=ORIENTED_EDGE('',*,*,#13473,.F.);
#17420=ORIENTED_EDGE('',*,*,#13474,.F.);
#17421=ORIENTED_EDGE('',*,*,#13471,.T.);
#17422=ORIENTED_EDGE('',*,*,#13475,.T.);
#17423=ORIENTED_EDGE('',*,*,#13445,.F.);
#17424=ORIENTED_EDGE('',*,*,#13447,.F.);
#17425=ORIENTED_EDGE('',*,*,#13450,.F.);
#17426=ORIENTED_EDGE('',*,*,#13453,.F.);
#17427=ORIENTED_EDGE('',*,*,#13456,.F.);
#17428=ORIENTED_EDGE('',*,*,#13459,.F.);
#17429=ORIENTED_EDGE('',*,*,#13462,.F.);
#17430=ORIENTED_EDGE('',*,*,#13464,.F.);
#17431=ORIENTED_EDGE('',*,*,#13476,.T.);
#17432=ORIENTED_EDGE('',*,*,#13477,.T.);
#17433=ORIENTED_EDGE('',*,*,#13478,.T.);
#17434=ORIENTED_EDGE('',*,*,#13479,.T.);
#17435=ORIENTED_EDGE('',*,*,#13480,.T.);
#17436=ORIENTED_EDGE('',*,*,#13481,.T.);
#17437=ORIENTED_EDGE('',*,*,#13482,.T.);
#17438=ORIENTED_EDGE('',*,*,#13483,.T.);
#17439=ORIENTED_EDGE('',*,*,#13484,.T.);
#17440=ORIENTED_EDGE('',*,*,#13474,.T.);
#17441=ORIENTED_EDGE('',*,*,#13485,.T.);
#17442=ORIENTED_EDGE('',*,*,#13486,.T.);
#17443=ORIENTED_EDGE('',*,*,#13487,.T.);
#17444=ORIENTED_EDGE('',*,*,#13488,.T.);
#17445=ORIENTED_EDGE('',*,*,#13485,.F.);
#17446=ORIENTED_EDGE('',*,*,#13489,.T.);
#17447=ORIENTED_EDGE('',*,*,#13490,.T.);
#17448=ORIENTED_EDGE('',*,*,#13491,.T.);
#17449=ORIENTED_EDGE('',*,*,#13487,.F.);
#17450=ORIENTED_EDGE('',*,*,#13492,.T.);
#17451=ORIENTED_EDGE('',*,*,#13493,.T.);
#17452=ORIENTED_EDGE('',*,*,#13494,.T.);
#17453=ORIENTED_EDGE('',*,*,#13490,.F.);
#17454=ORIENTED_EDGE('',*,*,#13495,.T.);
#17455=ORIENTED_EDGE('',*,*,#13496,.T.);
#17456=ORIENTED_EDGE('',*,*,#13497,.T.);
#17457=ORIENTED_EDGE('',*,*,#13493,.F.);
#17458=ORIENTED_EDGE('',*,*,#13498,.T.);
#17459=ORIENTED_EDGE('',*,*,#13499,.T.);
#17460=ORIENTED_EDGE('',*,*,#13500,.T.);
#17461=ORIENTED_EDGE('',*,*,#13496,.F.);
#17462=ORIENTED_EDGE('',*,*,#13467,.T.);
#17463=ORIENTED_EDGE('',*,*,#13501,.T.);
#17464=ORIENTED_EDGE('',*,*,#13502,.T.);
#17465=ORIENTED_EDGE('',*,*,#13499,.F.);
#17466=ORIENTED_EDGE('',*,*,#13470,.T.);
#17467=ORIENTED_EDGE('',*,*,#13501,.F.);
#17468=ORIENTED_EDGE('',*,*,#13472,.T.);
#17469=ORIENTED_EDGE('',*,*,#13484,.F.);
#17470=ORIENTED_EDGE('',*,*,#13503,.T.);
#17471=ORIENTED_EDGE('',*,*,#13460,.F.);
#17472=ORIENTED_EDGE('',*,*,#13504,.F.);
#17473=ORIENTED_EDGE('',*,*,#13495,.F.);
#17474=ORIENTED_EDGE('',*,*,#13505,.T.);
#17475=ORIENTED_EDGE('',*,*,#13463,.F.);
#17476=ORIENTED_EDGE('',*,*,#13505,.F.);
#17477=ORIENTED_EDGE('',*,*,#13492,.F.);
#17478=ORIENTED_EDGE('',*,*,#13506,.T.);
#17479=ORIENTED_EDGE('',*,*,#13465,.F.);
#17480=ORIENTED_EDGE('',*,*,#13506,.F.);
#17481=ORIENTED_EDGE('',*,*,#13489,.F.);
#17482=ORIENTED_EDGE('',*,*,#13473,.T.);
#17483=ORIENTED_EDGE('',*,*,#13486,.F.);
#17484=ORIENTED_EDGE('',*,*,#13488,.F.);
#17485=ORIENTED_EDGE('',*,*,#13491,.F.);
#17486=ORIENTED_EDGE('',*,*,#13494,.F.);
#17487=ORIENTED_EDGE('',*,*,#13497,.F.);
#17488=ORIENTED_EDGE('',*,*,#13500,.F.);
#17489=ORIENTED_EDGE('',*,*,#13502,.F.);
#17490=ORIENTED_EDGE('',*,*,#13503,.F.);
#17491=ORIENTED_EDGE('',*,*,#13507,.T.);
#17492=ORIENTED_EDGE('',*,*,#13508,.T.);
#17493=ORIENTED_EDGE('',*,*,#13509,.T.);
#17494=ORIENTED_EDGE('',*,*,#13510,.T.);
#17495=ORIENTED_EDGE('',*,*,#13511,.T.);
#17496=ORIENTED_EDGE('',*,*,#13512,.T.);
#17497=ORIENTED_EDGE('',*,*,#13513,.T.);
#17498=ORIENTED_EDGE('',*,*,#13514,.T.);
#17499=ORIENTED_EDGE('',*,*,#13476,.F.);
#17500=ORIENTED_EDGE('',*,*,#13515,.T.);
#17501=ORIENTED_EDGE('',*,*,#13516,.T.);
#17502=ORIENTED_EDGE('',*,*,#13515,.F.);
#17503=ORIENTED_EDGE('',*,*,#13516,.F.);
#17504=ORIENTED_EDGE('',*,*,#13477,.F.);
#17505=ORIENTED_EDGE('',*,*,#13517,.T.);
#17506=ORIENTED_EDGE('',*,*,#13518,.T.);
#17507=ORIENTED_EDGE('',*,*,#13517,.F.);
#17508=ORIENTED_EDGE('',*,*,#13518,.F.);
#17509=ORIENTED_EDGE('',*,*,#13507,.F.);
#17510=ORIENTED_EDGE('',*,*,#13519,.T.);
#17511=ORIENTED_EDGE('',*,*,#13520,.T.);
#17512=ORIENTED_EDGE('',*,*,#13519,.F.);
#17513=ORIENTED_EDGE('',*,*,#13520,.F.);
#17514=ORIENTED_EDGE('',*,*,#13508,.F.);
#17515=ORIENTED_EDGE('',*,*,#13521,.T.);
#17516=ORIENTED_EDGE('',*,*,#13522,.T.);
#17517=ORIENTED_EDGE('',*,*,#13521,.F.);
#17518=ORIENTED_EDGE('',*,*,#13522,.F.);
#17519=ORIENTED_EDGE('',*,*,#13514,.F.);
#17520=ORIENTED_EDGE('',*,*,#13523,.T.);
#17521=ORIENTED_EDGE('',*,*,#13483,.F.);
#17522=ORIENTED_EDGE('',*,*,#13523,.F.);
#17523=ORIENTED_EDGE('',*,*,#13513,.F.);
#17524=ORIENTED_EDGE('',*,*,#13524,.T.);
#17525=ORIENTED_EDGE('',*,*,#13482,.F.);
#17526=ORIENTED_EDGE('',*,*,#13524,.F.);
#17527=ORIENTED_EDGE('',*,*,#13512,.F.);
#17528=ORIENTED_EDGE('',*,*,#13525,.T.);
#17529=ORIENTED_EDGE('',*,*,#13481,.F.);
#17530=ORIENTED_EDGE('',*,*,#13525,.F.);
#17531=ORIENTED_EDGE('',*,*,#13511,.F.);
#17532=ORIENTED_EDGE('',*,*,#13526,.T.);
#17533=ORIENTED_EDGE('',*,*,#13480,.F.);
#17534=ORIENTED_EDGE('',*,*,#13526,.F.);
#17535=ORIENTED_EDGE('',*,*,#13527,.F.);
#17536=ORIENTED_EDGE('',*,*,#13528,.T.);
#17537=ORIENTED_EDGE('',*,*,#13529,.F.);
#17538=ORIENTED_EDGE('',*,*,#13530,.F.);
#17539=ORIENTED_EDGE('',*,*,#13531,.F.);
#17540=ORIENTED_EDGE('',*,*,#13528,.F.);
#17541=ORIENTED_EDGE('',*,*,#13529,.T.);
#17542=ORIENTED_EDGE('',*,*,#13531,.T.);
#17543=ORIENTED_EDGE('',*,*,#13532,.T.);
#17544=ORIENTED_EDGE('',*,*,#13478,.F.);
#17545=ORIENTED_EDGE('',*,*,#13533,.F.);
#17546=ORIENTED_EDGE('',*,*,#13534,.T.);
#17547=ORIENTED_EDGE('',*,*,#13535,.T.);
#17548=ORIENTED_EDGE('',*,*,#13536,.F.);
#17549=ORIENTED_EDGE('',*,*,#13509,.F.);
#17550=ORIENTED_EDGE('',*,*,#13537,.T.);
#17551=ORIENTED_EDGE('',*,*,#13440,.F.);
#17552=ORIENTED_EDGE('',*,*,#13527,.T.);
#17553=ORIENTED_EDGE('',*,*,#13538,.F.);
#17554=ORIENTED_EDGE('',*,*,#13539,.T.);
#17555=ORIENTED_EDGE('',*,*,#13441,.T.);
#17556=ORIENTED_EDGE('',*,*,#13539,.F.);
#17557=ORIENTED_EDGE('',*,*,#13540,.F.);
#17558=ORIENTED_EDGE('',*,*,#13541,.T.);
#17559=ORIENTED_EDGE('',*,*,#13534,.F.);
#17560=ORIENTED_EDGE('',*,*,#13542,.F.);
#17561=ORIENTED_EDGE('',*,*,#13535,.F.);
#17562=ORIENTED_EDGE('',*,*,#13541,.F.);
#17563=ORIENTED_EDGE('',*,*,#13530,.T.);
#17564=ORIENTED_EDGE('',*,*,#13537,.F.);
#17565=ORIENTED_EDGE('',*,*,#13510,.F.);
#17566=ORIENTED_EDGE('',*,*,#13536,.T.);
#17567=ORIENTED_EDGE('',*,*,#13542,.T.);
#17568=ORIENTED_EDGE('',*,*,#13533,.T.);
#17569=ORIENTED_EDGE('',*,*,#13479,.F.);
#17570=ORIENTED_EDGE('',*,*,#13532,.F.);
#17571=ORIENTED_EDGE('',*,*,#13434,.F.);
#17572=ORIENTED_EDGE('',*,*,#13540,.T.);
#17573=ORIENTED_EDGE('',*,*,#13475,.F.);
#17574=ORIENTED_EDGE('',*,*,#13543,.T.);
#17575=ORIENTED_EDGE('',*,*,#13435,.T.);
#17576=ORIENTED_EDGE('',*,*,#13543,.F.);
#17577=ORIENTED_EDGE('',*,*,#13457,.F.);
#17578=ORIENTED_EDGE('',*,*,#13468,.F.);
#17579=ORIENTED_EDGE('',*,*,#13498,.F.);
#17580=ORIENTED_EDGE('',*,*,#13504,.T.);
#17581=ORIENTED_EDGE('',*,*,#13538,.T.);
#23566=CONICAL_SURFACE('',#25446,13.8,0.785398163397448);
#23567=CONICAL_SURFACE('',#25453,13.8,0.785398163397448);
#23782=ADVANCED_FACE('',(#1923),#23566,.F.);
#23783=ADVANCED_FACE('',(#1924),#466,.F.);
#23784=ADVANCED_FACE('',(#1925,#611),#764,.T.);
#23785=ADVANCED_FACE('',(#1926),#23567,.F.);
#23786=ADVANCED_FACE('',(#1927),#467,.F.);
#23787=ADVANCED_FACE('',(#1928,#612),#765,.F.);
#23788=ADVANCED_FACE('',(#1929),#468,.T.);
#23789=ADVANCED_FACE('',(#1930),#225,.T.);
#23790=ADVANCED_FACE('',(#1931),#469,.T.);
#23791=ADVANCED_FACE('',(#1932),#226,.T.);
#23792=ADVANCED_FACE('',(#1933),#470,.T.);
#23793=ADVANCED_FACE('',(#1934),#227,.T.);
#23794=ADVANCED_FACE('',(#1935),#471,.T.);
#23795=ADVANCED_FACE('',(#1936),#228,.T.);
#23796=ADVANCED_FACE('',(#1937),#472,.T.);
#23797=ADVANCED_FACE('',(#1938),#766,.T.);
#23798=ADVANCED_FACE('',(#1939),#473,.T.);
#23799=ADVANCED_FACE('',(#1940,#613),#767,.T.);
#23800=ADVANCED_FACE('',(#1941,#614,#615,#616,#617,#618,#619,#620),#768,
 .T.);
#23801=ADVANCED_FACE('',(#1942),#474,.T.);
#23802=ADVANCED_FACE('',(#1943),#229,.T.);
#23803=ADVANCED_FACE('',(#1944),#475,.T.);
#23804=ADVANCED_FACE('',(#1945),#230,.T.);
#23805=ADVANCED_FACE('',(#1946),#476,.T.);
#23806=ADVANCED_FACE('',(#1947),#231,.T.);
#23807=ADVANCED_FACE('',(#1948),#477,.T.);
#23808=ADVANCED_FACE('',(#1949),#232,.T.);
#23809=ADVANCED_FACE('',(#1950),#478,.T.);
#23810=ADVANCED_FACE('',(#1951),#769,.T.);
#23811=ADVANCED_FACE('',(#1952),#479,.T.);
#23812=ADVANCED_FACE('',(#1953,#621,#622,#623,#624,#625,#626,#627),#770,
 .F.);
#23813=ADVANCED_FACE('',(#1954),#480,.F.);
#23814=ADVANCED_FACE('',(#1955),#771,.T.);
#23815=ADVANCED_FACE('',(#1956),#481,.F.);
#23816=ADVANCED_FACE('',(#1957),#772,.T.);
#23817=ADVANCED_FACE('',(#1958),#482,.F.);
#23818=ADVANCED_FACE('',(#1959),#773,.F.);
#23819=ADVANCED_FACE('',(#1960),#483,.F.);
#23820=ADVANCED_FACE('',(#1961),#774,.F.);
#23821=ADVANCED_FACE('',(#1962),#484,.F.);
#23822=ADVANCED_FACE('',(#1963),#485,.F.);
#23823=ADVANCED_FACE('',(#1964),#486,.F.);
#23824=ADVANCED_FACE('',(#1965),#487,.F.);
#23825=ADVANCED_FACE('',(#1966),#488,.F.);
#23826=ADVANCED_FACE('',(#1967),#489,.F.);
#23827=ADVANCED_FACE('',(#1968,#628),#775,.F.);
#23828=ADVANCED_FACE('',(#1969),#490,.F.);
#23829=ADVANCED_FACE('',(#1970),#491,.F.);
#23830=ADVANCED_FACE('',(#1971),#492,.F.);
#23831=ADVANCED_FACE('',(#1972,#629),#776,.T.);
#23832=ADVANCED_FACE('',(#1973),#493,.F.);
#23833=ADVANCED_FACE('',(#1974,#630),#777,.T.);
#24938=CLOSED_SHELL('',(#23782,#23783,#23784,#23785,#23786,#23787,#23788,
#23789,#23790,#23791,#23792,#23793,#23794,#23795,#23796,#23797,#23798,#23799,
#23800,#23801,#23802,#23803,#23804,#23805,#23806,#23807,#23808,#23809,#23810,
#23811,#23812,#23813,#23814,#23815,#23816,#23817,#23818,#23819,#23820,#23821,
#23822,#23823,#23824,#23825,#23826,#23827,#23828,#23829,#23830,#23831,#23832,
#23833));
#25445=AXIS2_PLACEMENT_3D('',#35319,#27799,#27800);
#25446=AXIS2_PLACEMENT_3D('',#35320,#27801,#27802);
#25447=AXIS2_PLACEMENT_3D('',#35322,#27803,#27804);
#25448=AXIS2_PLACEMENT_3D('',#35325,#27806,#27807);
#25449=AXIS2_PLACEMENT_3D('',#35326,#27808,#27809);
#25450=AXIS2_PLACEMENT_3D('',#35329,#27811,#27812);
#25451=AXIS2_PLACEMENT_3D('',#35330,#27813,#27814);
#25452=AXIS2_PLACEMENT_3D('',#35332,#27815,#27816);
#25453=AXIS2_PLACEMENT_3D('',#35333,#27817,#27818);
#25454=AXIS2_PLACEMENT_3D('',#35335,#27819,#27820);
#25455=AXIS2_PLACEMENT_3D('',#35338,#27822,#27823);
#25456=AXIS2_PLACEMENT_3D('',#35339,#27824,#27825);
#25457=AXIS2_PLACEMENT_3D('',#35342,#27827,#27828);
#25458=AXIS2_PLACEMENT_3D('',#35343,#27829,#27830);
#25459=AXIS2_PLACEMENT_3D('',#35345,#27831,#27832);
#25460=AXIS2_PLACEMENT_3D('',#35346,#27833,#27834);
#25461=AXIS2_PLACEMENT_3D('',#35349,#27835,#27836);
#25462=AXIS2_PLACEMENT_3D('',#35353,#27838,#27839);
#25463=AXIS2_PLACEMENT_3D('',#35355,#27841,#27842);
#25464=AXIS2_PLACEMENT_3D('',#35358,#27843,#27844);
#25465=AXIS2_PLACEMENT_3D('',#35359,#27845,#27846);
#25466=AXIS2_PLACEMENT_3D('',#35360,#27847,#27848);
#25467=AXIS2_PLACEMENT_3D('',#35361,#27849,#27850);
#25468=AXIS2_PLACEMENT_3D('',#35364,#27851,#27852);
#25469=AXIS2_PLACEMENT_3D('',#35367,#27855,#27856);
#25470=AXIS2_PLACEMENT_3D('',#35370,#27857,#27858);
#25471=AXIS2_PLACEMENT_3D('',#35371,#27859,#27860);
#25472=AXIS2_PLACEMENT_3D('',#35372,#27861,#27862);
#25473=AXIS2_PLACEMENT_3D('',#35373,#27863,#27864);
#25474=AXIS2_PLACEMENT_3D('',#35376,#27865,#27866);
#25475=AXIS2_PLACEMENT_3D('',#35379,#27869,#27870);
#25476=AXIS2_PLACEMENT_3D('',#35382,#27871,#27872);
#25477=AXIS2_PLACEMENT_3D('',#35383,#27873,#27874);
#25478=AXIS2_PLACEMENT_3D('',#35384,#27875,#27876);
#25479=AXIS2_PLACEMENT_3D('',#35385,#27877,#27878);
#25480=AXIS2_PLACEMENT_3D('',#35388,#27879,#27880);
#25481=AXIS2_PLACEMENT_3D('',#35391,#27883,#27884);
#25482=AXIS2_PLACEMENT_3D('',#35392,#27885,#27886);
#25483=AXIS2_PLACEMENT_3D('',#35393,#27887,#27888);
#25484=AXIS2_PLACEMENT_3D('',#35394,#27889,#27890);
#25485=AXIS2_PLACEMENT_3D('',#35398,#27892,#27893);
#25486=AXIS2_PLACEMENT_3D('',#35400,#27895,#27896);
#25487=AXIS2_PLACEMENT_3D('',#35404,#27899,#27900);
#25488=AXIS2_PLACEMENT_3D('',#35407,#27902,#27903);
#25489=AXIS2_PLACEMENT_3D('',#35408,#27904,#27905);
#25490=AXIS2_PLACEMENT_3D('',#35413,#27908,#27909);
#25491=AXIS2_PLACEMENT_3D('',#35414,#27910,#27911);
#25492=AXIS2_PLACEMENT_3D('',#35416,#27912,#27913);
#25493=AXIS2_PLACEMENT_3D('',#35418,#27914,#27915);
#25494=AXIS2_PLACEMENT_3D('',#35421,#27916,#27917);
#25495=AXIS2_PLACEMENT_3D('',#35422,#27918,#27919);
#25496=AXIS2_PLACEMENT_3D('',#35424,#27920,#27921);
#25497=AXIS2_PLACEMENT_3D('',#35426,#27922,#27923);
#25498=AXIS2_PLACEMENT_3D('',#35428,#27924,#27925);
#25499=AXIS2_PLACEMENT_3D('',#35430,#27926,#27927);
#25500=AXIS2_PLACEMENT_3D('',#35431,#27928,#27929);
#25501=AXIS2_PLACEMENT_3D('',#35433,#27930,#27931);
#25502=AXIS2_PLACEMENT_3D('',#35435,#27932,#27933);
#25503=AXIS2_PLACEMENT_3D('',#35437,#27935,#27936);
#25504=AXIS2_PLACEMENT_3D('',#35440,#27937,#27938);
#25505=AXIS2_PLACEMENT_3D('',#35441,#27939,#27940);
#25506=AXIS2_PLACEMENT_3D('',#35442,#27941,#27942);
#25507=AXIS2_PLACEMENT_3D('',#35443,#27943,#27944);
#25508=AXIS2_PLACEMENT_3D('',#35446,#27945,#27946);
#25509=AXIS2_PLACEMENT_3D('',#35449,#27949,#27950);
#25510=AXIS2_PLACEMENT_3D('',#35452,#27951,#27952);
#25511=AXIS2_PLACEMENT_3D('',#35453,#27953,#27954);
#25512=AXIS2_PLACEMENT_3D('',#35454,#27955,#27956);
#25513=AXIS2_PLACEMENT_3D('',#35455,#27957,#27958);
#25514=AXIS2_PLACEMENT_3D('',#35457,#27959,#27960);
#25515=AXIS2_PLACEMENT_3D('',#35460,#27963,#27964);
#25516=AXIS2_PLACEMENT_3D('',#35462,#27965,#27966);
#25517=AXIS2_PLACEMENT_3D('',#35463,#27967,#27968);
#25518=AXIS2_PLACEMENT_3D('',#35464,#27969,#27970);
#25519=AXIS2_PLACEMENT_3D('',#35466,#27971,#27972);
#25520=AXIS2_PLACEMENT_3D('',#35468,#27974,#27975);
#25521=AXIS2_PLACEMENT_3D('',#35469,#27976,#27977);
#25522=AXIS2_PLACEMENT_3D('',#35470,#27978,#27979);
#25523=AXIS2_PLACEMENT_3D('',#35473,#27982,#27983);
#25524=AXIS2_PLACEMENT_3D('',#35475,#27985,#27986);
#25525=AXIS2_PLACEMENT_3D('',#35476,#27987,#27988);
#25526=AXIS2_PLACEMENT_3D('',#35478,#27989,#27990);
#25527=AXIS2_PLACEMENT_3D('',#35480,#27991,#27992);
#25528=AXIS2_PLACEMENT_3D('',#35483,#27993,#27994);
#25529=AXIS2_PLACEMENT_3D('',#35484,#27995,#27996);
#25530=AXIS2_PLACEMENT_3D('',#35486,#27997,#27998);
#25531=AXIS2_PLACEMENT_3D('',#35488,#27999,#28000);
#25532=AXIS2_PLACEMENT_3D('',#35490,#28001,#28002);
#25533=AXIS2_PLACEMENT_3D('',#35492,#28003,#28004);
#25534=AXIS2_PLACEMENT_3D('',#35493,#28005,#28006);
#25535=AXIS2_PLACEMENT_3D('',#35496,#28008,#28009);
#25536=AXIS2_PLACEMENT_3D('',#35497,#28010,#28011);
#25537=AXIS2_PLACEMENT_3D('',#35498,#28012,#28013);
#25538=AXIS2_PLACEMENT_3D('',#35501,#28015,#28016);
#25539=AXIS2_PLACEMENT_3D('',#35502,#28017,#28018);
#25540=AXIS2_PLACEMENT_3D('',#35503,#28019,#28020);
#25541=AXIS2_PLACEMENT_3D('',#35506,#28022,#28023);
#25542=AXIS2_PLACEMENT_3D('',#35507,#28024,#28025);
#25543=AXIS2_PLACEMENT_3D('',#35508,#28026,#28027);
#25544=AXIS2_PLACEMENT_3D('',#35511,#28029,#28030);
#25545=AXIS2_PLACEMENT_3D('',#35512,#28031,#28032);
#25546=AXIS2_PLACEMENT_3D('',#35513,#28033,#28034);
#25547=AXIS2_PLACEMENT_3D('',#35515,#28036,#28037);
#25548=AXIS2_PLACEMENT_3D('',#35517,#28039,#28040);
#25549=AXIS2_PLACEMENT_3D('',#35519,#28042,#28043);
#25550=AXIS2_PLACEMENT_3D('',#35521,#28045,#28046);
#25551=AXIS2_PLACEMENT_3D('',#35523,#28047,#28048);
#25552=AXIS2_PLACEMENT_3D('',#35582,#28050,#28051);
#25553=AXIS2_PLACEMENT_3D('',#35618,#28056,#28057);
#25554=AXIS2_PLACEMENT_3D('',#35619,#28058,#28059);
#25555=AXIS2_PLACEMENT_3D('',#35621,#28060,#28061);
#25556=AXIS2_PLACEMENT_3D('',#35623,#28063,#28064);
#25557=AXIS2_PLACEMENT_3D('',#35625,#28065,#28066);
#25558=AXIS2_PLACEMENT_3D('',#35653,#28068,#28069);
#25559=AXIS2_PLACEMENT_3D('',#35654,#28070,#28071);
#25560=AXIS2_PLACEMENT_3D('',#35655,#28072,#28073);
#25561=AXIS2_PLACEMENT_3D('',#35657,#28075,#28076);
#27799=DIRECTION('axis',(0.,0.,1.));
#27800=DIRECTION('refdir',(1.,0.,0.));
#27801=DIRECTION('center_axis',(1.,0.,0.));
#27802=DIRECTION('ref_axis',(0.,0.,-1.));
#27803=DIRECTION('center_axis',(1.,0.,0.));
#27804=DIRECTION('ref_axis',(0.,0.,-1.));
#27805=DIRECTION('',(-0.707106781186547,8.65956056235493E-17,-0.707106781186547));
#27806=DIRECTION('center_axis',(-1.,0.,0.));
#27807=DIRECTION('ref_axis',(0.,0.,-1.));
#27808=DIRECTION('center_axis',(-1.,0.,0.));
#27809=DIRECTION('ref_axis',(0.,0.,-1.));
#27810=DIRECTION('',(-1.,0.,0.));
#27811=DIRECTION('center_axis',(-1.,0.,0.));
#27812=DIRECTION('ref_axis',(0.,0.,-1.));
#27813=DIRECTION('center_axis',(1.,0.,0.));
#27814=DIRECTION('ref_axis',(0.,0.,-1.));
#27815=DIRECTION('center_axis',(-1.,0.,0.));
#27816=DIRECTION('ref_axis',(0.,0.,-1.));
#27817=DIRECTION('center_axis',(-1.,0.,0.));
#27818=DIRECTION('ref_axis',(0.,0.,-1.));
#27819=DIRECTION('center_axis',(-1.,0.,0.));
#27820=DIRECTION('ref_axis',(0.,0.,-1.));
#27821=DIRECTION('',(0.707106781186547,-8.65956056235493E-17,-0.707106781186547));
#27822=DIRECTION('center_axis',(1.,0.,0.));
#27823=DIRECTION('ref_axis',(0.,0.,-1.));
#27824=DIRECTION('center_axis',(1.,0.,0.));
#27825=DIRECTION('ref_axis',(0.,0.,-1.));
#27826=DIRECTION('',(1.,0.,0.));
#27827=DIRECTION('center_axis',(1.,0.,0.));
#27828=DIRECTION('ref_axis',(0.,0.,-1.));
#27829=DIRECTION('center_axis',(1.,0.,0.));
#27830=DIRECTION('ref_axis',(0.,0.,-1.));
#27831=DIRECTION('center_axis',(1.,0.,0.));
#27832=DIRECTION('ref_axis',(0.,0.,-1.));
#27833=DIRECTION('center_axis',(0.,0.,-1.));
#27834=DIRECTION('ref_axis',(0.707106781186555,0.70710678118654,0.));
#27835=DIRECTION('center_axis',(0.,0.,-1.));
#27836=DIRECTION('ref_axis',(0.,1.,0.));
#27837=DIRECTION('',(0.,0.,-1.));
#27838=DIRECTION('center_axis',(0.,0.,1.));
#27839=DIRECTION('ref_axis',(1.,0.,0.));
#27840=DIRECTION('',(0.,0.,1.));
#27841=DIRECTION('center_axis',(0.,1.,0.));
#27842=DIRECTION('ref_axis',(0.,0.,1.));
#27843=DIRECTION('center_axis',(1.,0.,0.));
#27844=DIRECTION('ref_axis',(0.,0.,-1.));
#27845=DIRECTION('center_axis',(0.,-1.,0.));
#27846=DIRECTION('ref_axis',(0.707106781186548,0.,-0.707106781186548));
#27847=DIRECTION('center_axis',(0.,1.,0.));
#27848=DIRECTION('ref_axis',(0.707106781186548,0.,-0.707106781186548));
#27849=DIRECTION('center_axis',(-1.,0.,0.));
#27850=DIRECTION('ref_axis',(0.,0.70710678118654,-0.707106781186555));
#27851=DIRECTION('center_axis',(1.,0.,-5.55111512312578E-15));
#27852=DIRECTION('ref_axis',(-5.55111512312578E-15,0.,-1.));
#27853=DIRECTION('',(1.,0.,0.));
#27854=DIRECTION('',(-1.,0.,0.));
#27855=DIRECTION('center_axis',(0.,1.,0.));
#27856=DIRECTION('ref_axis',(0.,0.,1.));
#27857=DIRECTION('center_axis',(0.,0.,-1.));
#27858=DIRECTION('ref_axis',(-1.,0.,0.));
#27859=DIRECTION('center_axis',(0.,-1.,0.));
#27860=DIRECTION('ref_axis',(-0.707106781186547,0.,-0.707106781186548));
#27861=DIRECTION('center_axis',(0.,1.,0.));
#27862=DIRECTION('ref_axis',(-0.707106781186547,0.,-0.707106781186548));
#27863=DIRECTION('center_axis',(0.,0.,1.));
#27864=DIRECTION('ref_axis',(-0.707106781186555,0.70710678118654,0.));
#27865=DIRECTION('center_axis',(0.,0.,-1.));
#27866=DIRECTION('ref_axis',(-1.,0.,0.));
#27867=DIRECTION('',(0.,0.,-1.));
#27868=DIRECTION('',(0.,0.,1.));
#27869=DIRECTION('center_axis',(0.,1.,0.));
#27870=DIRECTION('ref_axis',(0.,0.,1.));
#27871=DIRECTION('center_axis',(-1.,0.,0.));
#27872=DIRECTION('ref_axis',(0.,0.,1.));
#27873=DIRECTION('center_axis',(0.,-1.,0.));
#27874=DIRECTION('ref_axis',(-0.707106781186548,0.,0.707106781186548));
#27875=DIRECTION('center_axis',(0.,1.,0.));
#27876=DIRECTION('ref_axis',(-0.707106781186548,0.,0.707106781186548));
#27877=DIRECTION('center_axis',(1.,0.,0.));
#27878=DIRECTION('ref_axis',(0.,0.70710678118654,0.707106781186555));
#27879=DIRECTION('center_axis',(-1.,0.,5.55111512312578E-15));
#27880=DIRECTION('ref_axis',(5.55111512312578E-15,0.,1.));
#27881=DIRECTION('',(-1.,0.,0.));
#27882=DIRECTION('',(1.,0.,0.));
#27883=DIRECTION('center_axis',(0.,1.,0.));
#27884=DIRECTION('ref_axis',(0.,0.,1.));
#27885=DIRECTION('center_axis',(0.,-1.,0.));
#27886=DIRECTION('ref_axis',(0.707106781186548,0.,0.707106781186548));
#27887=DIRECTION('center_axis',(0.,1.,0.));
#27888=DIRECTION('ref_axis',(0.707106781186548,0.,0.707106781186548));
#27889=DIRECTION('center_axis',(0.,1.,0.));
#27890=DIRECTION('ref_axis',(1.33226762955019E-15,0.,-1.));
#27891=DIRECTION('',(0.,1.,0.));
#27892=DIRECTION('center_axis',(0.,-1.,0.));
#27893=DIRECTION('ref_axis',(-0.707106781186547,0.,-0.707106781186548));
#27894=DIRECTION('',(0.,1.,0.));
#27895=DIRECTION('center_axis',(0.,0.,-1.));
#27896=DIRECTION('ref_axis',(-1.,0.,0.));
#27897=DIRECTION('',(0.,1.,0.));
#27898=DIRECTION('',(1.,0.,0.));
#27899=DIRECTION('center_axis',(0.,1.,0.));
#27900=DIRECTION('ref_axis',(1.,0.,8.88178419700126E-16));
#27901=DIRECTION('',(0.,1.,0.));
#27902=DIRECTION('center_axis',(0.,-1.,0.));
#27903=DIRECTION('ref_axis',(0.707106781186548,0.,-0.707106781186548));
#27904=DIRECTION('center_axis',(1.,0.,0.));
#27905=DIRECTION('ref_axis',(0.,0.,-1.));
#27906=DIRECTION('',(0.,1.,0.));
#27907=DIRECTION('',(0.,0.,1.));
#27908=DIRECTION('center_axis',(-1.,0.,0.));
#27909=DIRECTION('ref_axis',(0.,0.,-1.));
#27910=DIRECTION('center_axis',(0.,1.,0.));
#27911=DIRECTION('ref_axis',(1.,0.,0.));
#27912=DIRECTION('center_axis',(0.,-1.,0.));
#27913=DIRECTION('ref_axis',(1.,0.,0.));
#27914=DIRECTION('center_axis',(0.,-1.,0.));
#27915=DIRECTION('ref_axis',(1.,0.,0.));
#27916=DIRECTION('center_axis',(0.,-1.,0.));
#27917=DIRECTION('ref_axis',(1.,0.,0.));
#27918=DIRECTION('center_axis',(0.,-1.,0.));
#27919=DIRECTION('ref_axis',(1.,0.,0.));
#27920=DIRECTION('center_axis',(0.,-1.,0.));
#27921=DIRECTION('ref_axis',(1.,0.,0.));
#27922=DIRECTION('center_axis',(0.,-1.,0.));
#27923=DIRECTION('ref_axis',(1.,0.,0.));
#27924=DIRECTION('center_axis',(0.,-1.,0.));
#27925=DIRECTION('ref_axis',(1.,0.,0.));
#27926=DIRECTION('center_axis',(0.,-1.,0.));
#27927=DIRECTION('ref_axis',(1.,0.,0.));
#27928=DIRECTION('center_axis',(0.,0.,1.));
#27929=DIRECTION('ref_axis',(0.707106781186548,-0.707106781186548,0.));
#27930=DIRECTION('center_axis',(0.,0.,1.));
#27931=DIRECTION('ref_axis',(0.,-1.,0.));
#27932=DIRECTION('center_axis',(0.,0.,-1.));
#27933=DIRECTION('ref_axis',(1.,0.,0.));
#27934=DIRECTION('',(0.,0.,-1.));
#27935=DIRECTION('center_axis',(0.,1.,0.));
#27936=DIRECTION('ref_axis',(0.,0.,1.));
#27937=DIRECTION('center_axis',(1.,0.,0.));
#27938=DIRECTION('ref_axis',(0.,0.,1.));
#27939=DIRECTION('center_axis',(0.,1.,0.));
#27940=DIRECTION('ref_axis',(0.707106781186548,0.,0.707106781186548));
#27941=DIRECTION('center_axis',(0.,-1.,0.));
#27942=DIRECTION('ref_axis',(0.707106781186548,0.,0.707106781186548));
#27943=DIRECTION('center_axis',(-1.,0.,0.));
#27944=DIRECTION('ref_axis',(0.,-0.707106781186548,0.707106781186548));
#27945=DIRECTION('center_axis',(1.,0.,0.));
#27946=DIRECTION('ref_axis',(0.,0.,1.));
#27947=DIRECTION('',(1.,0.,0.));
#27948=DIRECTION('',(-1.,0.,0.));
#27949=DIRECTION('center_axis',(0.,1.,0.));
#27950=DIRECTION('ref_axis',(0.,0.,1.));
#27951=DIRECTION('center_axis',(5.55111512312581E-15,0.,1.));
#27952=DIRECTION('ref_axis',(-1.,0.,5.55111512312581E-15));
#27953=DIRECTION('center_axis',(0.,1.,0.));
#27954=DIRECTION('ref_axis',(-0.707106781186548,0.,0.707106781186548));
#27955=DIRECTION('center_axis',(0.,-1.,0.));
#27956=DIRECTION('ref_axis',(-0.707106781186548,0.,0.707106781186548));
#27957=DIRECTION('center_axis',(0.,0.,-1.));
#27958=DIRECTION('ref_axis',(-0.707106781186548,-0.707106781186548,0.));
#27959=DIRECTION('center_axis',(0.,0.,1.));
#27960=DIRECTION('ref_axis',(-1.,0.,0.));
#27961=DIRECTION('',(0.,0.,1.));
#27962=DIRECTION('',(0.,0.,-1.));
#27963=DIRECTION('center_axis',(0.,1.,0.));
#27964=DIRECTION('ref_axis',(0.,0.,1.));
#27965=DIRECTION('center_axis',(-1.,0.,-5.55111512312578E-15));
#27966=DIRECTION('ref_axis',(5.55111512312578E-15,0.,-1.));
#27967=DIRECTION('center_axis',(0.,1.,0.));
#27968=DIRECTION('ref_axis',(-0.707106781186547,0.,-0.707106781186548));
#27969=DIRECTION('center_axis',(1.,0.,0.));
#27970=DIRECTION('ref_axis',(0.,-0.707106781186548,-0.707106781186548));
#27971=DIRECTION('center_axis',(-1.,0.,0.));
#27972=DIRECTION('ref_axis',(0.,0.,-1.));
#27973=DIRECTION('',(-1.,0.,0.));
#27974=DIRECTION('center_axis',(0.,1.,0.));
#27975=DIRECTION('ref_axis',(0.,0.,1.));
#27976=DIRECTION('center_axis',(0.,1.,0.));
#27977=DIRECTION('ref_axis',(0.707106781186548,0.,-0.707106781186548));
#27978=DIRECTION('center_axis',(0.,1.,0.));
#27979=DIRECTION('ref_axis',(-1.,0.,-8.88178419700126E-16));
#27980=DIRECTION('',(0.,1.,0.));
#27981=DIRECTION('',(0.,1.,0.));
#27982=DIRECTION('center_axis',(0.,0.,1.));
#27983=DIRECTION('ref_axis',(1.,0.,0.));
#27984=DIRECTION('',(0.,1.,0.));
#27985=DIRECTION('center_axis',(0.,1.,0.));
#27986=DIRECTION('ref_axis',(-4.44089209850063E-16,0.,1.));
#27987=DIRECTION('center_axis',(0.,1.,0.));
#27988=DIRECTION('ref_axis',(1.,0.,0.));
#27989=DIRECTION('center_axis',(0.,1.,0.));
#27990=DIRECTION('ref_axis',(1.,0.,0.));
#27991=DIRECTION('center_axis',(0.,1.,0.));
#27992=DIRECTION('ref_axis',(1.,0.,0.));
#27993=DIRECTION('center_axis',(0.,1.,0.));
#27994=DIRECTION('ref_axis',(1.,0.,0.));
#27995=DIRECTION('center_axis',(0.,1.,0.));
#27996=DIRECTION('ref_axis',(1.,0.,0.));
#27997=DIRECTION('center_axis',(0.,1.,0.));
#27998=DIRECTION('ref_axis',(1.,0.,0.));
#27999=DIRECTION('center_axis',(0.,1.,0.));
#28000=DIRECTION('ref_axis',(1.,0.,0.));
#28001=DIRECTION('center_axis',(0.,1.,0.));
#28002=DIRECTION('ref_axis',(1.,0.,0.));
#28003=DIRECTION('center_axis',(0.,1.,0.));
#28004=DIRECTION('ref_axis',(1.,0.,0.));
#28005=DIRECTION('center_axis',(0.,-1.,0.));
#28006=DIRECTION('ref_axis',(1.,0.,0.));
#28007=DIRECTION('',(0.,-1.,0.));
#28008=DIRECTION('center_axis',(0.,-1.,0.));
#28009=DIRECTION('ref_axis',(1.,0.,0.));
#28010=DIRECTION('center_axis',(0.,1.,0.));
#28011=DIRECTION('ref_axis',(1.,0.,0.));
#28012=DIRECTION('center_axis',(0.,-1.,0.));
#28013=DIRECTION('ref_axis',(1.,0.,0.));
#28014=DIRECTION('',(0.,-1.,0.));
#28015=DIRECTION('center_axis',(0.,-1.,0.));
#28016=DIRECTION('ref_axis',(1.,0.,0.));
#28017=DIRECTION('center_axis',(0.,1.,0.));
#28018=DIRECTION('ref_axis',(1.,0.,0.));
#28019=DIRECTION('center_axis',(0.,1.,0.));
#28020=DIRECTION('ref_axis',(1.,0.,0.));
#28021=DIRECTION('',(0.,1.,0.));
#28022=DIRECTION('center_axis',(0.,1.,0.));
#28023=DIRECTION('ref_axis',(1.,0.,0.));
#28024=DIRECTION('center_axis',(0.,1.,0.));
#28025=DIRECTION('ref_axis',(1.,0.,0.));
#28026=DIRECTION('center_axis',(0.,1.,0.));
#28027=DIRECTION('ref_axis',(1.,0.,0.));
#28028=DIRECTION('',(0.,1.,0.));
#28029=DIRECTION('center_axis',(0.,1.,0.));
#28030=DIRECTION('ref_axis',(1.,0.,0.));
#28031=DIRECTION('center_axis',(0.,1.,0.));
#28032=DIRECTION('ref_axis',(1.,0.,0.));
#28033=DIRECTION('center_axis',(0.,1.,0.));
#28034=DIRECTION('ref_axis',(1.,0.,0.));
#28035=DIRECTION('',(0.,1.,0.));
#28036=DIRECTION('center_axis',(0.,1.,0.));
#28037=DIRECTION('ref_axis',(1.,0.,0.));
#28038=DIRECTION('',(0.,1.,0.));
#28039=DIRECTION('center_axis',(0.,1.,0.));
#28040=DIRECTION('ref_axis',(1.,0.,0.));
#28041=DIRECTION('',(0.,1.,0.));
#28042=DIRECTION('center_axis',(0.,1.,0.));
#28043=DIRECTION('ref_axis',(1.,0.,0.));
#28044=DIRECTION('',(0.,1.,0.));
#28045=DIRECTION('center_axis',(1.,0.,0.));
#28046=DIRECTION('ref_axis',(0.,0.,-1.));
#28047=DIRECTION('center_axis',(1.,0.,0.));
#28048=DIRECTION('ref_axis',(0.,0.,-1.));
#28049=DIRECTION('',(1.,0.,0.));
#28050=DIRECTION('center_axis',(0.,1.,0.));
#28051=DIRECTION('ref_axis',(-1.83697019872103E-16,0.,1.));
#28052=DIRECTION('',(0.,1.,0.));
#28053=DIRECTION('',(0.,1.,0.));
#28054=DIRECTION('',(0.,1.,0.));
#28055=DIRECTION('',(0.,1.,0.));
#28056=DIRECTION('center_axis',(1.,0.,0.));
#28057=DIRECTION('ref_axis',(0.,0.,-1.));
#28058=DIRECTION('center_axis',(1.,0.,0.));
#28059=DIRECTION('ref_axis',(0.,0.,-1.));
#28060=DIRECTION('center_axis',(1.,0.,0.));
#28061=DIRECTION('ref_axis',(0.,0.,-1.));
#28062=DIRECTION('',(1.,0.,0.));
#28063=DIRECTION('center_axis',(-1.,0.,0.));
#28064=DIRECTION('ref_axis',(0.,0.,-1.));
#28065=DIRECTION('center_axis',(-1.,0.,0.));
#28066=DIRECTION('ref_axis',(0.,0.,-1.));
#28067=DIRECTION('',(-1.,0.,0.));
#28068=DIRECTION('center_axis',(0.,1.,0.));
#28069=DIRECTION('ref_axis',(-1.83697019872103E-16,0.,-1.));
#28070=DIRECTION('center_axis',(1.,0.,0.));
#28071=DIRECTION('ref_axis',(0.,0.,-1.));
#28072=DIRECTION('center_axis',(-1.,0.,0.));
#28073=DIRECTION('ref_axis',(0.,0.,-1.));
#28074=DIRECTION('',(-1.,0.,0.));
#28075=DIRECTION('center_axis',(-1.,0.,0.));
#28076=DIRECTION('ref_axis',(0.,0.,1.));
#35319=CARTESIAN_POINT('',(0.,0.,0.));
#35320=CARTESIAN_POINT('Origin',(39.75,50.9,-16.5));
#35321=CARTESIAN_POINT('',(40.,50.9,-2.45));
#35322=CARTESIAN_POINT('Origin',(40.,50.9,-16.5));
#35323=CARTESIAN_POINT('',(39.5,50.9,-2.95));
#35324=CARTESIAN_POINT('',(39.75,50.9,-2.7));
#35325=CARTESIAN_POINT('Origin',(39.5,50.9,-16.5));
#35326=CARTESIAN_POINT('Origin',(40.,50.9,-16.5));
#35327=CARTESIAN_POINT('',(22.,50.9,-2.95));
#35328=CARTESIAN_POINT('',(40.,50.9,-2.95));
#35329=CARTESIAN_POINT('Origin',(22.,50.9,-16.5));
#35330=CARTESIAN_POINT('Origin',(40.,50.9,-16.5));
#35331=CARTESIAN_POINT('',(40.,50.9,4.5));
#35332=CARTESIAN_POINT('Origin',(40.,50.9,-16.5));
#35333=CARTESIAN_POINT('Origin',(-39.75,50.9,-16.5));
#35334=CARTESIAN_POINT('',(-40.,50.9,-2.45));
#35335=CARTESIAN_POINT('Origin',(-40.,50.9,-16.5));
#35336=CARTESIAN_POINT('',(-39.5,50.9,-2.95));
#35337=CARTESIAN_POINT('',(-39.75,50.9,-2.7));
#35338=CARTESIAN_POINT('Origin',(-39.5,50.9,-16.5));
#35339=CARTESIAN_POINT('Origin',(-40.,50.9,-16.5));
#35340=CARTESIAN_POINT('',(-22.,50.9,-2.95));
#35341=CARTESIAN_POINT('',(-40.,50.9,-2.95));
#35342=CARTESIAN_POINT('Origin',(-22.,50.9,-16.5));
#35343=CARTESIAN_POINT('Origin',(-40.,50.9,-16.5));
#35344=CARTESIAN_POINT('',(-40.,50.9,4.5));
#35345=CARTESIAN_POINT('Origin',(-40.,50.9,-16.5));
#35346=CARTESIAN_POINT('Origin',(39.7,83.2,4.25));
#35347=CARTESIAN_POINT('',(39.7,84.,25.));
#35348=CARTESIAN_POINT('',(40.5,83.2,25.));
#35349=CARTESIAN_POINT('Origin',(39.7,83.2,25.));
#35350=CARTESIAN_POINT('',(40.5,83.2,-58.));
#35351=CARTESIAN_POINT('',(40.5,83.2,4.25));
#35352=CARTESIAN_POINT('',(39.7,84.,-58.));
#35353=CARTESIAN_POINT('Origin',(39.7,83.2,-58.));
#35354=CARTESIAN_POINT('',(39.7,84.,4.25));
#35355=CARTESIAN_POINT('Origin',(30.5,83.2,-58.));
#35356=CARTESIAN_POINT('',(30.5,83.2,-68.));
#35357=CARTESIAN_POINT('',(30.5,84.,-67.2));
#35358=CARTESIAN_POINT('Origin',(30.5,83.2,-67.2));
#35359=CARTESIAN_POINT('Origin',(30.5,84.,-58.));
#35360=CARTESIAN_POINT('Origin',(30.5,83.2,-58.));
#35361=CARTESIAN_POINT('Origin',(15.25,83.2,-67.2));
#35362=CARTESIAN_POINT('',(-30.5,83.2,-68.));
#35363=CARTESIAN_POINT('',(-30.5,84.,-67.2));
#35364=CARTESIAN_POINT('Origin',(-30.5,83.2,-67.2));
#35365=CARTESIAN_POINT('',(15.25,84.,-67.2));
#35366=CARTESIAN_POINT('',(15.25,83.2,-68.));
#35367=CARTESIAN_POINT('Origin',(-30.5,83.2,-58.));
#35368=CARTESIAN_POINT('',(-40.5,83.2,-58.));
#35369=CARTESIAN_POINT('',(-39.7,84.,-58.));
#35370=CARTESIAN_POINT('Origin',(-39.7,83.2,-58.));
#35371=CARTESIAN_POINT('Origin',(-30.5,84.,-58.));
#35372=CARTESIAN_POINT('Origin',(-30.5,83.2,-58.));
#35373=CARTESIAN_POINT('Origin',(-39.7,83.2,-37.25));
#35374=CARTESIAN_POINT('',(-40.5,83.2,25.));
#35375=CARTESIAN_POINT('',(-39.7,84.,25.));
#35376=CARTESIAN_POINT('Origin',(-39.7,83.2,25.));
#35377=CARTESIAN_POINT('',(-39.7,84.,-37.25));
#35378=CARTESIAN_POINT('',(-40.5,83.2,-37.25));
#35379=CARTESIAN_POINT('Origin',(-30.5,83.2,25.));
#35380=CARTESIAN_POINT('',(-30.5,83.2,35.));
#35381=CARTESIAN_POINT('',(-30.5,84.,34.2));
#35382=CARTESIAN_POINT('Origin',(-30.5,83.2,34.2));
#35383=CARTESIAN_POINT('Origin',(-30.5,84.,25.));
#35384=CARTESIAN_POINT('Origin',(-30.5,83.2,25.));
#35385=CARTESIAN_POINT('Origin',(-15.25,83.2,34.2));
#35386=CARTESIAN_POINT('',(30.5,83.2,35.));
#35387=CARTESIAN_POINT('',(30.5,84.,34.2));
#35388=CARTESIAN_POINT('Origin',(30.5,83.2,34.2));
#35389=CARTESIAN_POINT('',(-15.25,84.,34.2));
#35390=CARTESIAN_POINT('',(-15.25,83.2,35.));
#35391=CARTESIAN_POINT('Origin',(30.5,83.2,25.));
#35392=CARTESIAN_POINT('Origin',(30.5,84.,25.));
#35393=CARTESIAN_POINT('Origin',(30.5,83.2,25.));
#35394=CARTESIAN_POINT('Origin',(-30.5,18.,-58.));
#35395=CARTESIAN_POINT('',(-30.5,18.8,-68.));
#35396=CARTESIAN_POINT('',(-30.5,18.,-68.));
#35397=CARTESIAN_POINT('',(-40.5,18.8,-58.));
#35398=CARTESIAN_POINT('Origin',(-30.5,18.8,-58.));
#35399=CARTESIAN_POINT('',(-40.5,18.,-58.));
#35400=CARTESIAN_POINT('Origin',(30.5,18.,-68.));
#35401=CARTESIAN_POINT('',(30.5,18.8,-68.));
#35402=CARTESIAN_POINT('',(30.5,18.,-68.));
#35403=CARTESIAN_POINT('',(15.25,18.8,-68.));
#35404=CARTESIAN_POINT('Origin',(30.5,18.,-58.));
#35405=CARTESIAN_POINT('',(40.5,18.8,-58.));
#35406=CARTESIAN_POINT('',(40.5,18.,-58.));
#35407=CARTESIAN_POINT('Origin',(30.5,18.8,-58.));
#35408=CARTESIAN_POINT('Origin',(40.5,18.,25.));
#35409=CARTESIAN_POINT('',(40.5,18.8,25.));
#35410=CARTESIAN_POINT('',(40.5,18.,25.));
#35411=CARTESIAN_POINT('',(40.5,18.8,4.25));
#35412=CARTESIAN_POINT('',(40.5,50.9,4.5));
#35413=CARTESIAN_POINT('Origin',(40.5,50.9,-16.5));
#35414=CARTESIAN_POINT('Origin',(0.,84.,-16.5));
#35415=CARTESIAN_POINT('',(26.49,84.,-16.5));
#35416=CARTESIAN_POINT('Origin',(30.5,84.,-16.5));
#35417=CARTESIAN_POINT('',(-34.51,84.,-16.5));
#35418=CARTESIAN_POINT('Origin',(-30.5,84.,-16.5));
#35419=CARTESIAN_POINT('',(10.0119928086271,84.,-16.5));
#35420=CARTESIAN_POINT('',(-10.0119928086271,84.,-16.5));
#35421=CARTESIAN_POINT('Origin',(0.,84.,0.));
#35422=CARTESIAN_POINT('Origin',(0.,84.,-33.));
#35423=CARTESIAN_POINT('',(-35.8,84.,-55.));
#35424=CARTESIAN_POINT('Origin',(-30.5,84.,-55.));
#35425=CARTESIAN_POINT('',(25.2,84.,22.));
#35426=CARTESIAN_POINT('Origin',(30.5,84.,22.));
#35427=CARTESIAN_POINT('',(-35.8,84.,22.));
#35428=CARTESIAN_POINT('Origin',(-30.5,84.,22.));
#35429=CARTESIAN_POINT('',(25.2,84.,-55.));
#35430=CARTESIAN_POINT('Origin',(30.5,84.,-55.));
#35431=CARTESIAN_POINT('Origin',(39.7,18.8,4.25));
#35432=CARTESIAN_POINT('',(39.7,18.,-58.));
#35433=CARTESIAN_POINT('Origin',(39.7,18.8,-58.));
#35434=CARTESIAN_POINT('',(39.7,18.,25.));
#35435=CARTESIAN_POINT('Origin',(39.7,18.8,25.));
#35436=CARTESIAN_POINT('',(39.7,18.,4.25));
#35437=CARTESIAN_POINT('Origin',(30.5,18.8,25.));
#35438=CARTESIAN_POINT('',(30.5,18.8,35.));
#35439=CARTESIAN_POINT('',(30.5,18.,34.2));
#35440=CARTESIAN_POINT('Origin',(30.5,18.8,34.2));
#35441=CARTESIAN_POINT('Origin',(30.5,18.,25.));
#35442=CARTESIAN_POINT('Origin',(30.5,18.8,25.));
#35443=CARTESIAN_POINT('Origin',(-15.25,18.8,34.2));
#35444=CARTESIAN_POINT('',(-30.5,18.8,35.));
#35445=CARTESIAN_POINT('',(-30.5,18.,34.2));
#35446=CARTESIAN_POINT('Origin',(-30.5,18.8,34.2));
#35447=CARTESIAN_POINT('',(-15.25,18.,34.2));
#35448=CARTESIAN_POINT('',(-15.25,18.8,35.));
#35449=CARTESIAN_POINT('Origin',(-30.5,18.8,25.));
#35450=CARTESIAN_POINT('',(-40.5,18.8,25.));
#35451=CARTESIAN_POINT('',(-39.7,18.,25.));
#35452=CARTESIAN_POINT('Origin',(-39.7,18.8,25.));
#35453=CARTESIAN_POINT('Origin',(-30.5,18.,25.));
#35454=CARTESIAN_POINT('Origin',(-30.5,18.8,25.));
#35455=CARTESIAN_POINT('Origin',(-39.7,18.8,-37.25));
#35456=CARTESIAN_POINT('',(-39.7,18.,-58.));
#35457=CARTESIAN_POINT('Origin',(-39.7,18.8,-58.));
#35458=CARTESIAN_POINT('',(-39.7,18.,-37.25));
#35459=CARTESIAN_POINT('',(-40.5,18.8,-37.25));
#35460=CARTESIAN_POINT('Origin',(-30.5,18.8,-58.));
#35461=CARTESIAN_POINT('',(-30.5,18.,-67.2));
#35462=CARTESIAN_POINT('Origin',(-30.5,18.8,-67.2));
#35463=CARTESIAN_POINT('Origin',(-30.5,18.,-58.));
#35464=CARTESIAN_POINT('Origin',(15.25,18.8,-67.2));
#35465=CARTESIAN_POINT('',(30.5,18.,-67.2));
#35466=CARTESIAN_POINT('Origin',(30.5,18.8,-67.2));
#35467=CARTESIAN_POINT('',(15.25,18.,-67.2));
#35468=CARTESIAN_POINT('Origin',(30.5,18.8,-58.));
#35469=CARTESIAN_POINT('Origin',(30.5,18.,-58.));
#35470=CARTESIAN_POINT('Origin',(-30.5,18.,25.));
#35471=CARTESIAN_POINT('',(-40.5,18.,25.));
#35472=CARTESIAN_POINT('',(-30.5,18.,35.));
#35473=CARTESIAN_POINT('Origin',(-30.5,18.,35.));
#35474=CARTESIAN_POINT('',(30.5,18.,35.));
#35475=CARTESIAN_POINT('Origin',(30.5,18.,25.));
#35476=CARTESIAN_POINT('Origin',(0.,18.,-16.5));
#35477=CARTESIAN_POINT('',(26.49,18.,-16.5));
#35478=CARTESIAN_POINT('Origin',(30.5,18.,-16.5));
#35479=CARTESIAN_POINT('',(-34.51,18.,-16.5));
#35480=CARTESIAN_POINT('Origin',(-30.5,18.,-16.5));
#35481=CARTESIAN_POINT('',(-10.0119928086271,18.,-16.5));
#35482=CARTESIAN_POINT('',(10.0119928086271,18.,-16.5));
#35483=CARTESIAN_POINT('Origin',(0.,18.,0.));
#35484=CARTESIAN_POINT('Origin',(0.,18.,-33.));
#35485=CARTESIAN_POINT('',(-35.8,18.,-55.));
#35486=CARTESIAN_POINT('Origin',(-30.5,18.,-55.));
#35487=CARTESIAN_POINT('',(25.2,18.,22.));
#35488=CARTESIAN_POINT('Origin',(30.5,18.,22.));
#35489=CARTESIAN_POINT('',(-35.8,18.,22.));
#35490=CARTESIAN_POINT('Origin',(-30.5,18.,22.));
#35491=CARTESIAN_POINT('',(25.2,18.,-55.));
#35492=CARTESIAN_POINT('Origin',(30.5,18.,-55.));
#35493=CARTESIAN_POINT('Origin',(30.5,84.,-16.5));
#35494=CARTESIAN_POINT('',(26.49,75.9,-16.5));
#35495=CARTESIAN_POINT('',(26.49,84.,-16.5));
#35496=CARTESIAN_POINT('Origin',(30.5,75.9,-16.5));
#35497=CARTESIAN_POINT('Origin',(30.5,75.9,-16.5));
#35498=CARTESIAN_POINT('Origin',(-30.5,84.,-16.5));
#35499=CARTESIAN_POINT('',(-34.51,75.9,-16.5));
#35500=CARTESIAN_POINT('',(-34.51,84.,-16.5));
#35501=CARTESIAN_POINT('Origin',(-30.5,75.9,-16.5));
#35502=CARTESIAN_POINT('Origin',(-30.5,75.9,-16.5));
#35503=CARTESIAN_POINT('Origin',(30.5,18.,-16.5));
#35504=CARTESIAN_POINT('',(26.49,26.1,-16.5));
#35505=CARTESIAN_POINT('',(26.49,18.,-16.5));
#35506=CARTESIAN_POINT('Origin',(30.5,26.1,-16.5));
#35507=CARTESIAN_POINT('Origin',(30.5,26.1,-16.5));
#35508=CARTESIAN_POINT('Origin',(-30.5,18.,-16.5));
#35509=CARTESIAN_POINT('',(-34.51,26.1,-16.5));
#35510=CARTESIAN_POINT('',(-34.51,18.,-16.5));
#35511=CARTESIAN_POINT('Origin',(-30.5,26.1,-16.5));
#35512=CARTESIAN_POINT('Origin',(-30.5,26.1,-16.5));
#35513=CARTESIAN_POINT('Origin',(30.5,18.,-55.));
#35514=CARTESIAN_POINT('',(25.2,18.,-55.));
#35515=CARTESIAN_POINT('Origin',(-30.5,18.,22.));
#35516=CARTESIAN_POINT('',(-35.8,18.,22.));
#35517=CARTESIAN_POINT('Origin',(30.5,18.,22.));
#35518=CARTESIAN_POINT('',(25.2,18.,22.));
#35519=CARTESIAN_POINT('Origin',(-30.5,18.,-55.));
#35520=CARTESIAN_POINT('',(-35.8,18.,-55.));
#35521=CARTESIAN_POINT('Origin',(-22.,50.9,-16.5));
#35522=CARTESIAN_POINT('',(-22.,50.9,-8.5));
#35523=CARTESIAN_POINT('Origin',(-22.,50.9,-16.5));
#35524=CARTESIAN_POINT('',(-17.3274348938324,50.9,-8.5));
#35525=CARTESIAN_POINT('',(-22.,50.9,-8.5));
#35526=CARTESIAN_POINT('',(-10.0119928086271,42.9,-16.5));
#35527=CARTESIAN_POINT('Ctrl Pts',(-10.0119928086271,42.9,-16.5));
#35528=CARTESIAN_POINT('Ctrl Pts',(-10.8243823748144,42.9,-16.0070522124563));
#35529=CARTESIAN_POINT('Ctrl Pts',(-11.5907592092305,42.9452825491298,-15.4594449915334));
#35530=CARTESIAN_POINT('Ctrl Pts',(-13.3968422560143,43.2558356261026,-13.965537209318));
#35531=CARTESIAN_POINT('Ctrl Pts',(-14.3590663403517,43.6180540935561,-12.9614726780539));
#35532=CARTESIAN_POINT('Ctrl Pts',(-15.5310939194137,44.6509559696764,-11.4729026436893));
#35533=CARTESIAN_POINT('Ctrl Pts',(-15.8830436339347,45.0733219142187,-10.9773729587387));
#35534=CARTESIAN_POINT('Ctrl Pts',(-16.4643944901793,46.0739061329322,-10.084517906201));
#35535=CARTESIAN_POINT('Ctrl Pts',(-16.6952841581299,46.6528137937707,-9.68893591004821));
#35536=CARTESIAN_POINT('Ctrl Pts',(-17.0124367279563,47.7580666714417,-9.1193277294487));
#35537=CARTESIAN_POINT('Ctrl Pts',(-17.1347583532058,48.3666931400295,-8.88370547669544));
#35538=CARTESIAN_POINT('Ctrl Pts',(-17.2918616244663,49.6341178547131,-8.57389564467795));
#35539=CARTESIAN_POINT('Ctrl Pts',(-17.3274348938324,50.2928891954098,-8.5));
#35540=CARTESIAN_POINT('Ctrl Pts',(-17.3274348938324,50.9,-8.5));
#35541=CARTESIAN_POINT('',(-10.0119928086271,58.9,-16.5));
#35542=CARTESIAN_POINT('Ctrl Pts',(-10.0119928086271,58.9,-16.5));
#35543=CARTESIAN_POINT('Ctrl Pts',(-10.8243823748144,58.9,-16.9929477875437));
#35544=CARTESIAN_POINT('Ctrl Pts',(-11.5907592092305,58.8547174508702,-17.5405550084666));
#35545=CARTESIAN_POINT('Ctrl Pts',(-13.3968422560143,58.5441643738974,-19.034462790682));
#35546=CARTESIAN_POINT('Ctrl Pts',(-14.3590663403517,58.1819459064439,-20.0385273219461));
#35547=CARTESIAN_POINT('Ctrl Pts',(-15.5310939194137,57.1490440303236,-21.5270973563107));
#35548=CARTESIAN_POINT('Ctrl Pts',(-15.8830436339347,56.7266780857813,-22.0226270412612));
#35549=CARTESIAN_POINT('Ctrl Pts',(-16.4643944901793,55.7260938670678,-22.915482093799));
#35550=CARTESIAN_POINT('Ctrl Pts',(-16.6952841581299,55.1471862062293,-23.3110640899518));
#35551=CARTESIAN_POINT('Ctrl Pts',(-17.0124367279563,54.0419333285583,-23.8806722705513));
#35552=CARTESIAN_POINT('Ctrl Pts',(-17.1347583532058,53.4333068599705,-24.1162945233046));
#35553=CARTESIAN_POINT('Ctrl Pts',(-17.2918616244663,52.1658821452869,-24.4261043553221));
#35554=CARTESIAN_POINT('Ctrl Pts',(-17.3274348938324,51.5071108045901,-24.5));
#35555=CARTESIAN_POINT('Ctrl Pts',(-17.3274348938324,50.2928891954098,-24.5));
#35556=CARTESIAN_POINT('Ctrl Pts',(-17.2918616244663,49.6341178547131,-24.4261043553221));
#35557=CARTESIAN_POINT('Ctrl Pts',(-17.1347583532058,48.3666931400295,-24.1162945233046));
#35558=CARTESIAN_POINT('Ctrl Pts',(-17.0124367279563,47.7580666714417,-23.8806722705513));
#35559=CARTESIAN_POINT('Ctrl Pts',(-16.6952841581299,46.6528137937707,-23.3110640899518));
#35560=CARTESIAN_POINT('Ctrl Pts',(-16.4643944901793,46.0739061329322,-22.915482093799));
#35561=CARTESIAN_POINT('Ctrl Pts',(-15.8830436339347,45.0733219142187,-22.0226270412612));
#35562=CARTESIAN_POINT('Ctrl Pts',(-15.5310939194137,44.6509559696764,-21.5270973563107));
#35563=CARTESIAN_POINT('Ctrl Pts',(-14.3590663403517,43.6180540935561,-20.0385273219461));
#35564=CARTESIAN_POINT('Ctrl Pts',(-13.3968422560143,43.2558356261026,-19.034462790682));
#35565=CARTESIAN_POINT('Ctrl Pts',(-11.5907592092305,42.9452825491298,-17.5405550084666));
#35566=CARTESIAN_POINT('Ctrl Pts',(-10.8243823748144,42.9,-16.9929477875437));
#35567=CARTESIAN_POINT('Ctrl Pts',(-10.0119928086271,42.9,-16.5));
#35568=CARTESIAN_POINT('Ctrl Pts',(-17.3274348938324,50.9,-8.5));
#35569=CARTESIAN_POINT('Ctrl Pts',(-17.3274348938324,51.5071108045902,-8.5));
#35570=CARTESIAN_POINT('Ctrl Pts',(-17.2918616244663,52.1658821452869,-8.57389564467795));
#35571=CARTESIAN_POINT('Ctrl Pts',(-17.1347583532058,53.4333068599705,-8.88370547669544));
#35572=CARTESIAN_POINT('Ctrl Pts',(-17.0124367279563,54.0419333285583,-9.1193277294487));
#35573=CARTESIAN_POINT('Ctrl Pts',(-16.6952841581299,55.1471862062293,-9.68893591004821));
#35574=CARTESIAN_POINT('Ctrl Pts',(-16.4643944901793,55.7260938670678,-10.084517906201));
#35575=CARTESIAN_POINT('Ctrl Pts',(-15.8830436339347,56.7266780857813,-10.9773729587387));
#35576=CARTESIAN_POINT('Ctrl Pts',(-15.5310939194137,57.1490440303236,-11.4729026436893));
#35577=CARTESIAN_POINT('Ctrl Pts',(-14.3590663403517,58.1819459064439,-12.9614726780539));
#35578=CARTESIAN_POINT('Ctrl Pts',(-13.3968422560143,58.5441643738974,-13.965537209318));
#35579=CARTESIAN_POINT('Ctrl Pts',(-11.5907592092305,58.8547174508702,-15.4594449915334));
#35580=CARTESIAN_POINT('Ctrl Pts',(-10.8243823748144,58.9,-16.0070522124563));
#35581=CARTESIAN_POINT('Ctrl Pts',(-10.0119928086271,58.9,-16.5));
#35582=CARTESIAN_POINT('Origin',(0.,18.,0.));
#35583=CARTESIAN_POINT('',(-10.0119928086271,18.,-16.5));
#35584=CARTESIAN_POINT('',(10.0119928086271,58.9,-16.5));
#35585=CARTESIAN_POINT('',(10.0119928086271,18.,-16.5));
#35586=CARTESIAN_POINT('',(17.3274348938324,50.9,-8.5));
#35587=CARTESIAN_POINT('Ctrl Pts',(10.0119928086271,58.9,-16.5));
#35588=CARTESIAN_POINT('Ctrl Pts',(10.8243823748144,58.9,-16.0070522124563));
#35589=CARTESIAN_POINT('Ctrl Pts',(11.5907592092305,58.8547174508702,-15.4594449915334));
#35590=CARTESIAN_POINT('Ctrl Pts',(13.3968422560143,58.5441643738974,-13.965537209318));
#35591=CARTESIAN_POINT('Ctrl Pts',(14.3590663403517,58.1819459064439,-12.9614726780539));
#35592=CARTESIAN_POINT('Ctrl Pts',(15.5310939194137,57.1490440303236,-11.4729026436893));
#35593=CARTESIAN_POINT('Ctrl Pts',(15.8830436339347,56.7266780857813,-10.9773729587387));
#35594=CARTESIAN_POINT('Ctrl Pts',(16.4643944901793,55.7260938670678,-10.084517906201));
#35595=CARTESIAN_POINT('Ctrl Pts',(16.6952841581299,55.1471862062293,-9.68893591004821));
#35596=CARTESIAN_POINT('Ctrl Pts',(17.0124367279563,54.0419333285583,-9.1193277294487));
#35597=CARTESIAN_POINT('Ctrl Pts',(17.1347583532058,53.4333068599705,-8.88370547669544));
#35598=CARTESIAN_POINT('Ctrl Pts',(17.2918616244663,52.1658821452869,-8.57389564467795));
#35599=CARTESIAN_POINT('Ctrl Pts',(17.3274348938324,51.5071108045902,-8.5));
#35600=CARTESIAN_POINT('Ctrl Pts',(17.3274348938324,50.9,-8.5));
#35601=CARTESIAN_POINT('',(10.0119928086271,42.9,-16.5));
#35602=CARTESIAN_POINT('Ctrl Pts',(17.3274348938324,50.9,-8.5));
#35603=CARTESIAN_POINT('Ctrl Pts',(17.3274348938324,50.2928891954098,-8.5));
#35604=CARTESIAN_POINT('Ctrl Pts',(17.2918616244663,49.6341178547131,-8.57389564467795));
#35605=CARTESIAN_POINT('Ctrl Pts',(17.1347583532058,48.3666931400295,-8.88370547669544));
#35606=CARTESIAN_POINT('Ctrl Pts',(17.0124367279563,47.7580666714417,-9.1193277294487));
#35607=CARTESIAN_POINT('Ctrl Pts',(16.6952841581299,46.6528137937707,-9.68893591004821));
#35608=CARTESIAN_POINT('Ctrl Pts',(16.4643944901793,46.0739061329322,-10.084517906201));
#35609=CARTESIAN_POINT('Ctrl Pts',(15.8830436339347,45.0733219142187,-10.9773729587387));
#35610=CARTESIAN_POINT('Ctrl Pts',(15.5310939194137,44.6509559696764,-11.4729026436893));
#35611=CARTESIAN_POINT('Ctrl Pts',(14.3590663403517,43.6180540935561,-12.9614726780539));
#35612=CARTESIAN_POINT('Ctrl Pts',(13.3968422560143,43.2558356261026,-13.965537209318));
#35613=CARTESIAN_POINT('Ctrl Pts',(11.5907592092305,42.9452825491298,-15.4594449915334));
#35614=CARTESIAN_POINT('Ctrl Pts',(10.8243823748144,42.9,-16.0070522124563));
#35615=CARTESIAN_POINT('Ctrl Pts',(10.0119928086271,42.9,-16.5));
#35616=CARTESIAN_POINT('',(10.0119928086271,18.,-16.5));
#35617=CARTESIAN_POINT('',(-10.0119928086271,18.,-16.5));
#35618=CARTESIAN_POINT('Origin',(-22.,50.9,-16.5));
#35619=CARTESIAN_POINT('Origin',(-40.5,50.9,-16.5));
#35620=CARTESIAN_POINT('',(-40.5,50.9,4.5));
#35621=CARTESIAN_POINT('Origin',(-40.5,50.9,-16.5));
#35622=CARTESIAN_POINT('',(-40.5,50.9,4.5));
#35623=CARTESIAN_POINT('Origin',(22.,50.9,-16.5));
#35624=CARTESIAN_POINT('',(22.,50.9,-8.5));
#35625=CARTESIAN_POINT('Origin',(22.,50.9,-16.5));
#35626=CARTESIAN_POINT('',(22.,50.9,-8.5));
#35627=CARTESIAN_POINT('Ctrl Pts',(10.0119928086271,42.9,-16.5));
#35628=CARTESIAN_POINT('Ctrl Pts',(10.8243823748144,42.9,-16.9929477875437));
#35629=CARTESIAN_POINT('Ctrl Pts',(11.5907592092305,42.9452825491298,-17.5405550084666));
#35630=CARTESIAN_POINT('Ctrl Pts',(13.3968422560143,43.2558356261026,-19.034462790682));
#35631=CARTESIAN_POINT('Ctrl Pts',(14.3590663403517,43.6180540935561,-20.0385273219461));
#35632=CARTESIAN_POINT('Ctrl Pts',(15.5310939194137,44.6509559696764,-21.5270973563107));
#35633=CARTESIAN_POINT('Ctrl Pts',(15.8830436339347,45.0733219142187,-22.0226270412612));
#35634=CARTESIAN_POINT('Ctrl Pts',(16.4643944901793,46.0739061329322,-22.915482093799));
#35635=CARTESIAN_POINT('Ctrl Pts',(16.6952841581299,46.6528137937707,-23.3110640899518));
#35636=CARTESIAN_POINT('Ctrl Pts',(17.0124367279563,47.7580666714417,-23.8806722705513));
#35637=CARTESIAN_POINT('Ctrl Pts',(17.1347583532058,48.3666931400295,-24.1162945233046));
#35638=CARTESIAN_POINT('Ctrl Pts',(17.2918616244663,49.6341178547131,-24.4261043553221));
#35639=CARTESIAN_POINT('Ctrl Pts',(17.3274348938324,50.2928891954098,-24.5));
#35640=CARTESIAN_POINT('Ctrl Pts',(17.3274348938324,51.5071108045901,-24.5));
#35641=CARTESIAN_POINT('Ctrl Pts',(17.2918616244663,52.1658821452869,-24.4261043553221));
#35642=CARTESIAN_POINT('Ctrl Pts',(17.1347583532058,53.4333068599705,-24.1162945233046));
#35643=CARTESIAN_POINT('Ctrl Pts',(17.0124367279563,54.0419333285583,-23.8806722705513));
#35644=CARTESIAN_POINT('Ctrl Pts',(16.6952841581299,55.1471862062293,-23.3110640899518));
#35645=CARTESIAN_POINT('Ctrl Pts',(16.4643944901793,55.7260938670678,-22.915482093799));
#35646=CARTESIAN_POINT('Ctrl Pts',(15.8830436339347,56.7266780857813,-22.0226270412612));
#35647=CARTESIAN_POINT('Ctrl Pts',(15.5310939194137,57.1490440303236,-21.5270973563107));
#35648=CARTESIAN_POINT('Ctrl Pts',(14.3590663403517,58.1819459064439,-20.0385273219461));
#35649=CARTESIAN_POINT('Ctrl Pts',(13.3968422560143,58.5441643738974,-19.034462790682));
#35650=CARTESIAN_POINT('Ctrl Pts',(11.5907592092305,58.8547174508702,-17.5405550084666));
#35651=CARTESIAN_POINT('Ctrl Pts',(10.8243823748144,58.9,-16.9929477875437));
#35652=CARTESIAN_POINT('Ctrl Pts',(10.0119928086271,58.9,-16.5));
#35653=CARTESIAN_POINT('Origin',(0.,18.,-33.));
#35654=CARTESIAN_POINT('Origin',(22.,50.9,-16.5));
#35655=CARTESIAN_POINT('Origin',(40.5,50.9,-16.5));
#35656=CARTESIAN_POINT('',(40.5,50.9,4.5));
#35657=CARTESIAN_POINT('Origin',(-40.5,18.,-58.));
#46366=UNCERTAINTY_MEASURE_WITH_UNIT(LENGTH_MEASURE(0.01),#46396,
'DISTANCE_ACCURACY_VALUE',
'Maximum model space distance between geometric entities at asserted c
onnectivities');
#46379=UNCERTAINTY_MEASURE_WITH_UNIT(LENGTH_MEASURE(0.01),#46396,
'DISTANCE_ACCURACY_VALUE',
'Maximum model space distance between geometric entities at asserted c
onnectivities');
#46382=(
GEOMETRIC_REPRESENTATION_CONTEXT(3)
GLOBAL_UNCERTAINTY_ASSIGNED_CONTEXT((#46366))
GLOBAL_UNIT_ASSIGNED_CONTEXT((#46396,#46398,#46399))
REPRESENTATION_CONTEXT('','3D')
);
#46395=(
GEOMETRIC_REPRESENTATION_CONTEXT(3)
GLOBAL_UNCERTAINTY_ASSIGNED_CONTEXT((#46379))
GLOBAL_UNIT_ASSIGNED_CONTEXT((#46396,#46398,#46399))
REPRESENTATION_CONTEXT('','3D')
);
#46396=(
LENGTH_UNIT()
NAMED_UNIT(*)
SI_UNIT(.MILLI.,.METRE.)
);
#46398=(
NAMED_UNIT(*)
PLANE_ANGLE_UNIT()
SI_UNIT($,.RADIAN.)
);
#46399=(
NAMED_UNIT(*)
SI_UNIT($,.STERADIAN.)
SOLID_ANGLE_UNIT()
);
#46402=SHAPE_DEFINITION_REPRESENTATION(#46417,#46457);
#46417=PRODUCT_DEFINITION_SHAPE('',$,#46473);
#46457=SHAPE_REPRESENTATION('',(#25445),#46382);
#46470=PRODUCT_DEFINITION_CONTEXT('part definition',#46517,'design');
#46473=PRODUCT_DEFINITION('2026-10-26-00-50-40-883','02_Gear_Body',#46488,
#46470);
#46488=PRODUCT_DEFINITION_FORMATION('',$,#46521);
#46517=APPLICATION_CONTEXT(
'Core Data for Automotive Mechanical Design Process');
#46518=PRODUCT_CONTEXT('part definition',#46517,'mechanical');
#46521=PRODUCT('2026-10-26-00-50-40-883','02_Gear_Body',$,(#46518));
#46569=COLOUR_RGB('Dark Blue',0.08,0.2,0.34);
#46570=FILL_AREA_STYLE_COLOUR('',#46569);
#46571=FILL_AREA_STYLE('',(#46570));
#46572=SURFACE_STYLE_FILL_AREA(#46571);
#46573=SURFACE_SIDE_STYLE('',(#46572));
#46574=SURFACE_STYLE_USAGE(.BOTH.,#46573);
#46575=PRESENTATION_STYLE_ASSIGNMENT((#46574));
ENDSEC;
END-ISO-10303-21;
